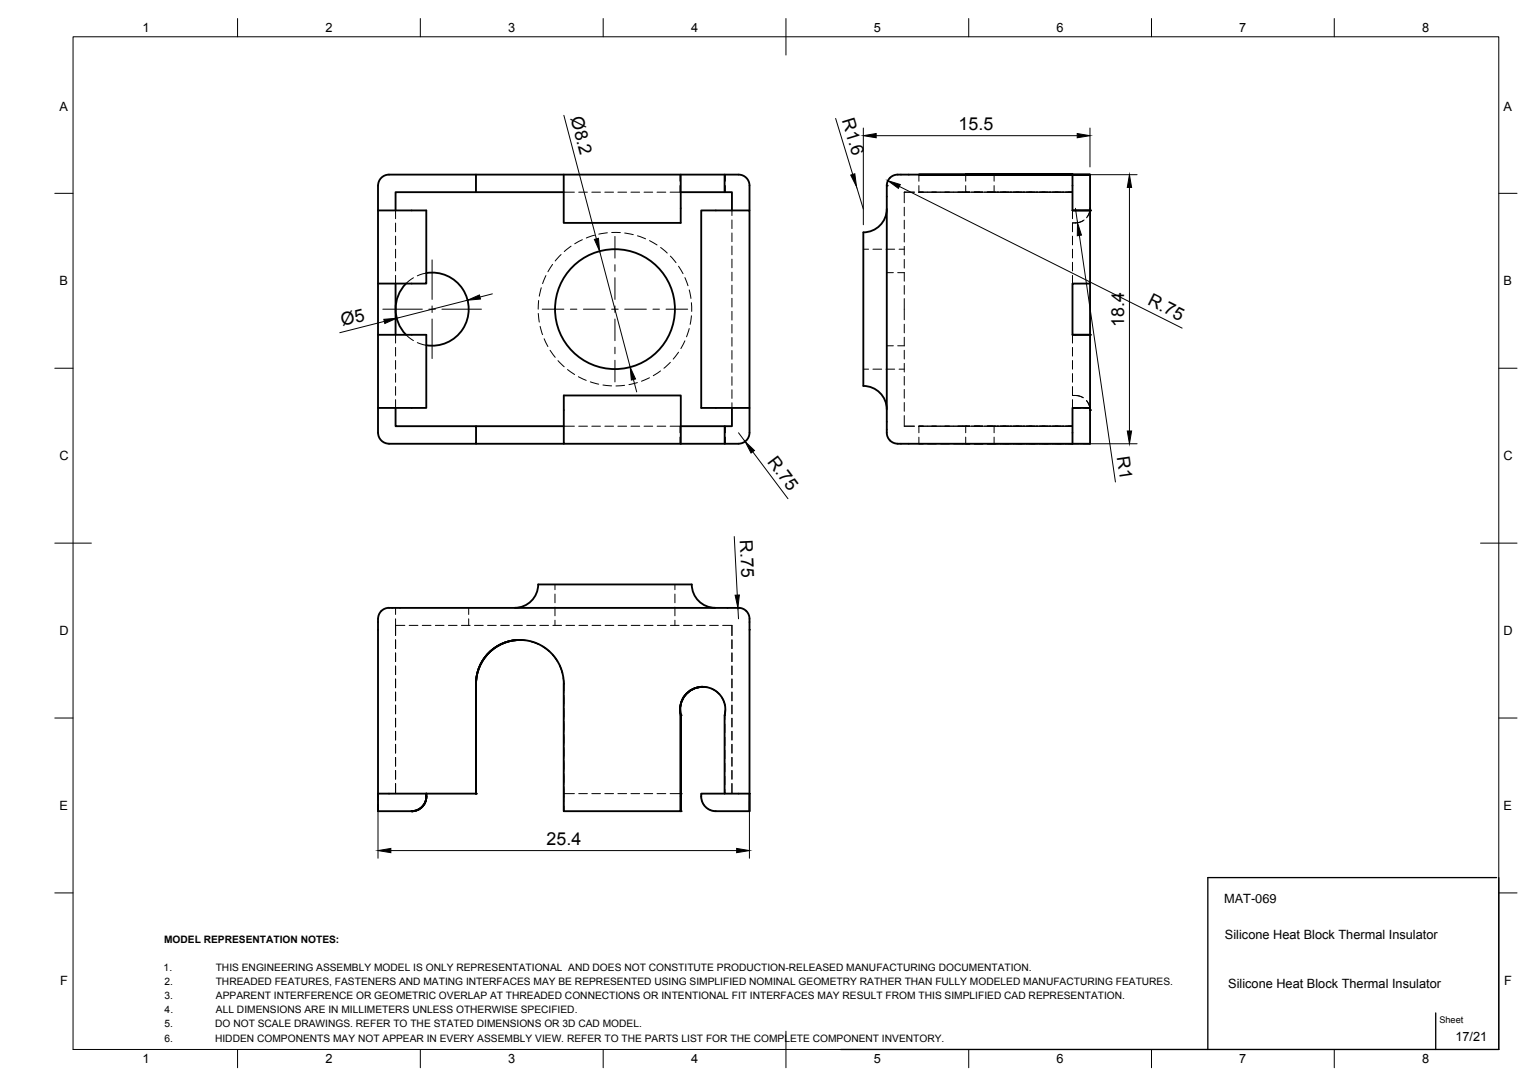
ISO-10303-21;
HEADER;
/* Generated by software containing ST-Developer
 * from STEP Tools, Inc. (www.steptools.com) 
 */

FILE_DESCRIPTION(
/* description */ ('CAx-IF Rec.Pracs.---Representation and Presentation of Product Manufa
cturing Information (PMI)---4.0---2014-10-13'),
/* implementation_level */ '2;1');

FILE_NAME(
/* name */ 'Silicone Heat Block Thermal Insulator.step',
/* time_stamp */ '2026-10-24T15:08:39-07:00',
/* author */ (''),
/* organization */ (''),
/* preprocessor_version */ 'ST-DEVELOPER v20.2',
/* originating_system */ 'Autodesk Translation Framework v15.17.0.0',
/* authorisation */ '');

FILE_SCHEMA (('AP242_MANAGED_MODEL_BASED_3D_ENGINEERING_MIM_LF { 1 0 10303 442 2 1 4 }'));
ENDSEC;

DATA;
#10=MECHANICAL_DESIGN_GEOMETRIC_PRESENTATION_REPRESENTATION('',(#834),#50081);
#115=B_SPLINE_SURFACE_WITH_KNOTS('',3,3,((#44428,#44429,#44430,#44431,#44432,
#44433),(#44434,#44435,#44436,#44437,#44438,#44439),(#44440,#44441,#44442,
#44443,#44444,#44445),(#44446,#44447,#44448,#44449,#44450,#44451),(#44452,
#44453,#44454,#44455,#44456,#44457),(#44458,#44459,#44460,#44461,#44462,
#44463)),.UNSPECIFIED.,.F.,.F.,.F.,(4,1,1,4),(4,1,1,4),(0.,0.333333333333333,
0.666666666666667,1.00005609897907),(-5.60989790777921E-5,0.333333333333333,
0.666666666666667,1.00005609897908),.UNSPECIFIED.);
#116=B_SPLINE_SURFACE_WITH_KNOTS('',3,3,((#44482,#44483,#44484,#44485,#44486,
#44487),(#44488,#44489,#44490,#44491,#44492,#44493),(#44494,#44495,#44496,
#44497,#44498,#44499),(#44500,#44501,#44502,#44503,#44504,#44505),(#44506,
#44507,#44508,#44509,#44510,#44511),(#44512,#44513,#44514,#44515,#44516,
#44517)),.UNSPECIFIED.,.F.,.F.,.F.,(4,1,1,4),(4,1,1,4),(-5.60989790420212E-5,
0.333333333333333,0.666666666666667,1.00005609897904),(0.,0.333333333333333,
0.666666666666667,1.00005609897904),.UNSPECIFIED.);
#117=B_SPLINE_SURFACE_WITH_KNOTS('',3,3,((#44528,#44529,#44530,#44531,#44532,
#44533),(#44534,#44535,#44536,#44537,#44538,#44539),(#44540,#44541,#44542,
#44543,#44544,#44545),(#44546,#44547,#44548,#44549,#44550,#44551),(#44552,
#44553,#44554,#44555,#44556,#44557),(#44558,#44559,#44560,#44561,#44562,
#44563)),.UNSPECIFIED.,.F.,.F.,.F.,(4,1,1,4),(4,1,1,4),(0.,0.333333333333333,
0.666666666666667,1.00005609897908),(-5.60989790915146E-5,0.333333333333333,
0.666666666666667,1.00005609897909),.UNSPECIFIED.);
#118=B_SPLINE_SURFACE_WITH_KNOTS('',3,3,((#44574,#44575,#44576,#44577,#44578,
#44579),(#44580,#44581,#44582,#44583,#44584,#44585),(#44586,#44587,#44588,
#44589,#44590,#44591),(#44592,#44593,#44594,#44595,#44596,#44597),(#44598,
#44599,#44600,#44601,#44602,#44603),(#44604,#44605,#44606,#44607,#44608,
#44609)),.UNSPECIFIED.,.F.,.F.,.F.,(4,1,1,4),(4,1,1,4),(-5.60989790792135E-5,
0.333333333333333,0.666666666666667,1.00005609897908),(0.,0.333333333333333,
0.666666666666667,1.00005609897907),.UNSPECIFIED.);
#119=B_SPLINE_SURFACE_WITH_KNOTS('',3,3,((#44620,#44621,#44622,#44623,#44624,
#44625),(#44626,#44627,#44628,#44629,#44630,#44631),(#44632,#44633,#44634,
#44635,#44636,#44637),(#44638,#44639,#44640,#44641,#44642,#44643),(#44644,
#44645,#44646,#44647,#44648,#44649),(#44650,#44651,#44652,#44653,#44654,
#44655)),.UNSPECIFIED.,.F.,.F.,.F.,(4,1,1,4),(4,1,1,4),(0.,0.333333333333333,
0.666666666666667,1.00005609897905),(-5.60989790491253E-5,0.333333333333333,
0.666666666666667,1.00005609897905),.UNSPECIFIED.);
#120=B_SPLINE_SURFACE_WITH_KNOTS('',3,3,((#44666,#44667,#44668,#44669,#44670,
#44671),(#44672,#44673,#44674,#44675,#44676,#44677),(#44678,#44679,#44680,
#44681,#44682,#44683),(#44684,#44685,#44686,#44687,#44688,#44689),(#44690,
#44691,#44692,#44693,#44694,#44695),(#44696,#44697,#44698,#44699,#44700,
#44701)),.UNSPECIFIED.,.F.,.F.,.F.,(4,1,1,4),(4,1,1,4),(0.,0.333333333333333,
0.666666666666667,1.00005609897395),(-5.60989810489178E-5,0.333333333333333,
0.666666666666667,1.00005609898105),.UNSPECIFIED.);
#121=B_SPLINE_SURFACE_WITH_KNOTS('',3,3,((#44720,#44721,#44722,#44723,#44724,
#44725),(#44726,#44727,#44728,#44729,#44730,#44731),(#44732,#44733,#44734,
#44735,#44736,#44737),(#44738,#44739,#44740,#44741,#44742,#44743),(#44744,
#44745,#44746,#44747,#44748,#44749),(#44750,#44751,#44752,#44753,#44754,
#44755)),.UNSPECIFIED.,.F.,.F.,.F.,(4,1,1,4),(4,1,1,4),(-5.60989793261701E-5,
0.333333333333333,0.666666666666667,1.00005609897933),(0.,0.333333333333333,
0.666666666666667,1.00005609896406),.UNSPECIFIED.);
#122=B_SPLINE_SURFACE_WITH_KNOTS('',3,3,((#44766,#44767,#44768,#44769,#44770,
#44771),(#44772,#44773,#44774,#44775,#44776,#44777),(#44778,#44779,#44780,
#44781,#44782,#44783),(#44784,#44785,#44786,#44787,#44788,#44789),(#44790,
#44791,#44792,#44793,#44794,#44795),(#44796,#44797,#44798,#44799,#44800,
#44801)),.UNSPECIFIED.,.F.,.F.,.F.,(4,1,1,4),(4,1,1,4),(0.,0.333333333333333,
0.666666666666667,1.00005609897906),(-5.60989790758371E-5,0.333333333333333,
0.666666666666667,1.00005609897907),.UNSPECIFIED.);
#123=B_SPLINE_SURFACE_WITH_KNOTS('',3,3,((#44812,#44813,#44814,#44815,#44816,
#44817),(#44818,#44819,#44820,#44821,#44822,#44823),(#44824,#44825,#44826,
#44827,#44828,#44829),(#44830,#44831,#44832,#44833,#44834,#44835),(#44836,
#44837,#44838,#44839,#44840,#44841),(#44842,#44843,#44844,#44845,#44846,
#44847)),.UNSPECIFIED.,.F.,.F.,.F.,(4,1,1,4),(4,1,1,4),(-5.60989790925808E-5,
0.333333333333333,0.666666666666667,1.00005609897909),(0.,0.333333333333333,
0.666666666666667,1.00005609897908),.UNSPECIFIED.);
#124=B_SPLINE_SURFACE_WITH_KNOTS('',3,3,((#44858,#44859,#44860,#44861,#44862,
#44863),(#44864,#44865,#44866,#44867,#44868,#44869),(#44870,#44871,#44872,
#44873,#44874,#44875),(#44876,#44877,#44878,#44879,#44880,#44881),(#44882,
#44883,#44884,#44885,#44886,#44887),(#44888,#44889,#44890,#44891,#44892,
#44893)),.UNSPECIFIED.,.F.,.F.,.F.,(4,1,1,4),(4,1,1,4),(0.,0.333333333333333,
0.666666666666667,1.00005609896405),(-5.60989793186213E-5,0.333333333333333,
0.666666666666667,1.00005609897932),.UNSPECIFIED.);
#125=B_SPLINE_SURFACE_WITH_KNOTS('',3,3,((#44904,#44905,#44906,#44907,#44908,
#44909),(#44910,#44911,#44912,#44913,#44914,#44915),(#44916,#44917,#44918,
#44919,#44920,#44921),(#44922,#44923,#44924,#44925,#44926,#44927),(#44928,
#44929,#44930,#44931,#44932,#44933),(#44934,#44935,#44936,#44937,#44938,
#44939)),.UNSPECIFIED.,.F.,.F.,.F.,(4,1,1,4),(4,1,1,4),(0.,0.333333333333333,
0.666666666666667,1.00005609896408),(-5.60989793518835E-5,0.333333333333333,
0.666666666666667,1.00005609897935),.UNSPECIFIED.);
#126=B_SPLINE_SURFACE_WITH_KNOTS('',3,3,((#44958,#44959,#44960,#44961,#44962,
#44963),(#44964,#44965,#44966,#44967,#44968,#44969),(#44970,#44971,#44972,
#44973,#44974,#44975),(#44976,#44977,#44978,#44979,#44980,#44981),(#44982,
#44983,#44984,#44985,#44986,#44987),(#44988,#44989,#44990,#44991,#44992,
#44993)),.UNSPECIFIED.,.F.,.F.,.F.,(4,1,1,4),(4,1,1,4),(-5.60989810425424E-5,
0.333333333333333,0.666666666666667,1.00005609898105),(0.,0.333333333333333,
0.666666666666667,1.00005609897395),.UNSPECIFIED.);
#127=B_SPLINE_SURFACE_WITH_KNOTS('',3,3,((#45004,#45005,#45006,#45007,#45008,
#45009),(#45010,#45011,#45012,#45013,#45014,#45015),(#45016,#45017,#45018,
#45019,#45020,#45021),(#45022,#45023,#45024,#45025,#45026,#45027),(#45028,
#45029,#45030,#45031,#45032,#45033),(#45034,#45035,#45036,#45037,#45038,
#45039)),.UNSPECIFIED.,.F.,.F.,.F.,(4,1,1,4),(4,1,1,4),(0.,0.333333333333333,
0.666666666666667,1.00005609897391),(-5.60989809954259E-5,0.333333333333333,
0.666666666666667,1.000056098981),.UNSPECIFIED.);
#128=B_SPLINE_SURFACE_WITH_KNOTS('',3,3,((#45050,#45051,#45052,#45053,#45054,
#45055),(#45056,#45057,#45058,#45059,#45060,#45061),(#45062,#45063,#45064,
#45065,#45066,#45067),(#45068,#45069,#45070,#45071,#45072,#45073),(#45074,
#45075,#45076,#45077,#45078,#45079),(#45080,#45081,#45082,#45083,#45084,
#45085)),.UNSPECIFIED.,.F.,.F.,.F.,(4,1,1,4),(4,1,1,4),(-5.60989793233286E-5,
0.333333333333333,0.666666666666667,1.00005609897932),(0.,0.333333333333333,
0.666666666666667,1.00005609896406),.UNSPECIFIED.);
#129=B_SPLINE_SURFACE_WITH_KNOTS('',3,3,((#45096,#45097,#45098,#45099,#45100,
#45101),(#45102,#45103,#45104,#45105,#45106,#45107),(#45108,#45109,#45110,
#45111,#45112,#45113),(#45114,#45115,#45116,#45117,#45118,#45119),(#45120,
#45121,#45122,#45123,#45124,#45125),(#45126,#45127,#45128,#45129,#45130,
#45131)),.UNSPECIFIED.,.F.,.F.,.F.,(4,1,1,4),(4,1,1,4),(0.,0.333333333333333,
0.666666666666667,1.0000560989791),(-5.60989791002414E-5,0.333333333333333,
0.666666666666667,1.0000560989791),.UNSPECIFIED.);
#130=B_SPLINE_SURFACE_WITH_KNOTS('',3,3,((#45142,#45143,#45144,#45145,#45146,
#45147),(#45148,#45149,#45150,#45151,#45152,#45153),(#45154,#45155,#45156,
#45157,#45158,#45159),(#45160,#45161,#45162,#45163,#45164,#45165),(#45166,
#45167,#45168,#45169,#45170,#45171),(#45172,#45173,#45174,#45175,#45176,
#45177)),.UNSPECIFIED.,.F.,.F.,.F.,(4,1,1,4),(4,1,1,4),(0.,0.333333333333333,
0.666666666666667,1.00005609896409),(-5.60989793533921E-5,0.333333333333333,
0.666666666666667,1.00005609897935),.UNSPECIFIED.);
#131=B_SPLINE_SURFACE_WITH_KNOTS('',3,3,((#45196,#45197,#45198,#45199,#45200,
#45201),(#45202,#45203,#45204,#45205,#45206,#45207),(#45208,#45209,#45210,
#45211,#45212,#45213),(#45214,#45215,#45216,#45217,#45218,#45219),(#45220,
#45221,#45222,#45223,#45224,#45225),(#45226,#45227,#45228,#45229,#45230,
#45231)),.UNSPECIFIED.,.F.,.F.,.F.,(4,1,1,4),(4,1,1,4),(-5.60989810493619E-5,
0.333333333333333,0.666666666666667,1.00005609898105),(0.,0.333333333333333,
0.666666666666667,1.00005609897395),.UNSPECIFIED.);
#132=B_SPLINE_SURFACE_WITH_KNOTS('',3,3,((#45242,#45243,#45244,#45245,#45246,
#45247),(#45248,#45249,#45250,#45251,#45252,#45253),(#45254,#45255,#45256,
#45257,#45258,#45259),(#45260,#45261,#45262,#45263,#45264,#45265),(#45266,
#45267,#45268,#45269,#45270,#45271),(#45272,#45273,#45274,#45275,#45276,
#45277)),.UNSPECIFIED.,.F.,.F.,.F.,(4,1,1,4),(4,1,1,4),(0.,0.333333333333333,
0.666666666666667,1.00005609895074),(-5.60989812701836E-5,0.333333333333333,
0.666666666666667,1.00005609898127),.UNSPECIFIED.);
#133=B_SPLINE_SURFACE_WITH_KNOTS('',3,3,((#45288,#45289,#45290,#45291,#45292,
#45293),(#45294,#45295,#45296,#45297,#45298,#45299),(#45300,#45301,#45302,
#45303,#45304,#45305),(#45306,#45307,#45308,#45309,#45310,#45311),(#45312,
#45313,#45314,#45315,#45316,#45317),(#45318,#45319,#45320,#45321,#45322,
#45323)),.UNSPECIFIED.,.F.,.F.,.F.,(4,1,1,4),(4,1,1,4),(-5.60989812733151E-5,
0.333333333333333,0.666666666666667,1.00005609898127),(0.,0.333333333333333,
0.666666666666667,1.00005609895075),.UNSPECIFIED.);
#134=B_SPLINE_SURFACE_WITH_KNOTS('',3,3,((#45334,#45335,#45336,#45337,#45338,
#45339),(#45340,#45341,#45342,#45343,#45344,#45345),(#45346,#45347,#45348,
#45349,#45350,#45351),(#45352,#45353,#45354,#45355,#45356,#45357),(#45358,
#45359,#45360,#45361,#45362,#45363),(#45364,#45365,#45366,#45367,#45368,
#45369)),.UNSPECIFIED.,.F.,.F.,.F.,(4,1,1,4),(4,1,1,4),(0.,0.333333333333333,
0.666666666666667,1.00005609897395),(-5.60989810488734E-5,0.333333333333333,
0.666666666666667,1.00005609898105),.UNSPECIFIED.);
#135=B_SPLINE_SURFACE_WITH_KNOTS('',3,3,((#45380,#45381,#45382,#45383,#45384,
#45385),(#45386,#45387,#45388,#45389,#45390,#45391),(#45392,#45393,#45394,
#45395,#45396,#45397),(#45398,#45399,#45400,#45401,#45402,#45403),(#45404,
#45405,#45406,#45407,#45408,#45409),(#45410,#45411,#45412,#45413,#45414,
#45415)),.UNSPECIFIED.,.F.,.F.,.F.,(4,1,1,4),(4,1,1,4),(-5.60989793545037E-5,
0.333333333333333,0.666666666666667,1.00005609897935),(0.,0.333333333333333,
0.666666666666667,1.00005609896409),.UNSPECIFIED.);
#136=B_SPLINE_SURFACE_WITH_KNOTS('',3,3,((#45425,#45426,#45427,#45428,#45429,
#45430),(#45431,#45432,#45433,#45434,#45435,#45436),(#45437,#45438,#45439,
#45440,#45441,#45442),(#45443,#45444,#45445,#45446,#45447,#45448),(#45449,
#45450,#45451,#45452,#45453,#45454),(#45455,#45456,#45457,#45458,#45459,
#45460)),.UNSPECIFIED.,.F.,.F.,.F.,(4,1,1,4),(4,1,1,4),(-5.60989790782798E-5,
0.333333333333333,0.666666666666667,1.00005609897908),(0.,0.333333333333333,
0.666666666666667,1.00005609897908),.UNSPECIFIED.);
#137=B_SPLINE_SURFACE_WITH_KNOTS('',3,3,((#45473,#45474,#45475,#45476,#45477,
#45478),(#45479,#45480,#45481,#45482,#45483,#45484),(#45485,#45486,#45487,
#45488,#45489,#45490),(#45491,#45492,#45493,#45494,#45495,#45496),(#45497,
#45498,#45499,#45500,#45501,#45502),(#45503,#45504,#45505,#45506,#45507,
#45508)),.UNSPECIFIED.,.F.,.F.,.F.,(4,1,1,4),(4,1,1,4),(-5.60989810261355E-5,
0.333333333333333,0.666666666666667,1.00005609898103),(0.,0.333333333333333,
0.666666666666667,1.00005609897399),.UNSPECIFIED.);
#138=B_SPLINE_SURFACE_WITH_KNOTS('',3,3,((#45518,#45519,#45520,#45521,#45522,
#45523),(#45524,#45525,#45526,#45527,#45528,#45529),(#45530,#45531,#45532,
#45533,#45534,#45535),(#45536,#45537,#45538,#45539,#45540,#45541),(#45542,
#45543,#45544,#45545,#45546,#45547),(#45548,#45549,#45550,#45551,#45552,
#45553)),.UNSPECIFIED.,.F.,.F.,.F.,(4,1,1,4),(4,1,1,4),(-5.6098979101063E-5,
0.333333333333333,0.666666666666667,1.0000560989791),(0.,0.333333333333333,
0.666666666666667,1.0000560989791),.UNSPECIFIED.);
#493=B_SPLINE_CURVE_WITH_KNOTS('',3,(#44466,#44467,#44468,#44469,#44470,
#44471),.UNSPECIFIED.,.F.,.F.,(4,1,1,4),(0.,0.333333333333333,0.666666666666667,
1.),.UNSPECIFIED.);
#494=B_SPLINE_CURVE_WITH_KNOTS('',3,(#44473,#44474,#44475,#44476,#44477,
#44478),.UNSPECIFIED.,.F.,.F.,(4,1,1,4),(0.,0.333333333333333,0.666666666666667,
1.),.UNSPECIFIED.);
#495=B_SPLINE_CURVE_WITH_KNOTS('',3,(#44519,#44520,#44521,#44522,#44523,
#44524),.UNSPECIFIED.,.F.,.F.,(4,1,1,4),(0.,0.333333333333333,0.666666666666667,
1.),.UNSPECIFIED.);
#496=B_SPLINE_CURVE_WITH_KNOTS('',3,(#44565,#44566,#44567,#44568,#44569,
#44570),.UNSPECIFIED.,.F.,.F.,(4,1,1,4),(0.,0.333333333333333,0.666666666666667,
1.),.UNSPECIFIED.);
#497=B_SPLINE_CURVE_WITH_KNOTS('',3,(#44611,#44612,#44613,#44614,#44615,
#44616),.UNSPECIFIED.,.F.,.F.,(4,1,1,4),(0.,0.333333333333333,0.666666666666667,
1.),.UNSPECIFIED.);
#498=B_SPLINE_CURVE_WITH_KNOTS('',3,(#44657,#44658,#44659,#44660,#44661,
#44662),.UNSPECIFIED.,.F.,.F.,(4,1,1,4),(0.,0.333333333333333,0.666666666666667,
1.),.UNSPECIFIED.);
#499=B_SPLINE_CURVE_WITH_KNOTS('',3,(#44704,#44705,#44706,#44707,#44708,
#44709),.UNSPECIFIED.,.F.,.F.,(4,1,1,4),(0.,0.333333333333333,0.666666666666667,
1.),.UNSPECIFIED.);
#500=B_SPLINE_CURVE_WITH_KNOTS('',3,(#44711,#44712,#44713,#44714,#44715,
#44716),.UNSPECIFIED.,.F.,.F.,(4,1,1,4),(0.,0.333333333333333,0.666666666666667,
1.),.UNSPECIFIED.);
#501=B_SPLINE_CURVE_WITH_KNOTS('',3,(#44757,#44758,#44759,#44760,#44761,
#44762),.UNSPECIFIED.,.F.,.F.,(4,1,1,4),(0.,0.333333333333333,0.666666666666667,
1.),.UNSPECIFIED.);
#502=B_SPLINE_CURVE_WITH_KNOTS('',3,(#44803,#44804,#44805,#44806,#44807,
#44808),.UNSPECIFIED.,.F.,.F.,(4,1,1,4),(0.,0.333333333333333,0.666666666666667,
1.),.UNSPECIFIED.);
#503=B_SPLINE_CURVE_WITH_KNOTS('',3,(#44849,#44850,#44851,#44852,#44853,
#44854),.UNSPECIFIED.,.F.,.F.,(4,1,1,4),(0.,0.333333333333333,0.666666666666667,
1.),.UNSPECIFIED.);
#504=B_SPLINE_CURVE_WITH_KNOTS('',3,(#44895,#44896,#44897,#44898,#44899,
#44900),.UNSPECIFIED.,.F.,.F.,(4,1,1,4),(0.,0.333333333333333,0.666666666666667,
1.),.UNSPECIFIED.);
#505=B_SPLINE_CURVE_WITH_KNOTS('',3,(#44942,#44943,#44944,#44945,#44946,
#44947),.UNSPECIFIED.,.F.,.F.,(4,1,1,4),(0.,0.333333333333333,0.666666666666667,
1.),.UNSPECIFIED.);
#506=B_SPLINE_CURVE_WITH_KNOTS('',3,(#44949,#44950,#44951,#44952,#44953,
#44954),.UNSPECIFIED.,.F.,.F.,(4,1,1,4),(0.,0.333333333333333,0.666666666666667,
1.),.UNSPECIFIED.);
#507=B_SPLINE_CURVE_WITH_KNOTS('',3,(#44995,#44996,#44997,#44998,#44999,
#45000),.UNSPECIFIED.,.F.,.F.,(4,1,1,4),(0.,0.333333333333333,0.666666666666667,
1.),.UNSPECIFIED.);
#508=B_SPLINE_CURVE_WITH_KNOTS('',3,(#45041,#45042,#45043,#45044,#45045,
#45046),.UNSPECIFIED.,.F.,.F.,(4,1,1,4),(0.,0.333333333333333,0.666666666666667,
1.),.UNSPECIFIED.);
#509=B_SPLINE_CURVE_WITH_KNOTS('',3,(#45087,#45088,#45089,#45090,#45091,
#45092),.UNSPECIFIED.,.F.,.F.,(4,1,1,4),(0.,0.333333333333333,0.666666666666667,
1.),.UNSPECIFIED.);
#510=B_SPLINE_CURVE_WITH_KNOTS('',3,(#45133,#45134,#45135,#45136,#45137,
#45138),.UNSPECIFIED.,.F.,.F.,(4,1,1,4),(0.,0.333333333333333,0.666666666666667,
1.),.UNSPECIFIED.);
#511=B_SPLINE_CURVE_WITH_KNOTS('',3,(#45180,#45181,#45182,#45183,#45184,
#45185),.UNSPECIFIED.,.F.,.F.,(4,1,1,4),(0.,0.333333333333333,0.666666666666667,
1.),.UNSPECIFIED.);
#512=B_SPLINE_CURVE_WITH_KNOTS('',3,(#45187,#45188,#45189,#45190,#45191,
#45192),.UNSPECIFIED.,.F.,.F.,(4,1,1,4),(0.,0.333333333333333,0.666666666666667,
1.),.UNSPECIFIED.);
#513=B_SPLINE_CURVE_WITH_KNOTS('',3,(#45233,#45234,#45235,#45236,#45237,
#45238),.UNSPECIFIED.,.F.,.F.,(4,1,1,4),(0.,0.333333333333333,0.666666666666667,
1.),.UNSPECIFIED.);
#514=B_SPLINE_CURVE_WITH_KNOTS('',3,(#45279,#45280,#45281,#45282,#45283,
#45284),.UNSPECIFIED.,.F.,.F.,(4,1,1,4),(0.,0.333333333333333,0.666666666666667,
1.),.UNSPECIFIED.);
#515=B_SPLINE_CURVE_WITH_KNOTS('',3,(#45325,#45326,#45327,#45328,#45329,
#45330),.UNSPECIFIED.,.F.,.F.,(4,1,1,4),(0.,0.333333333333333,0.666666666666667,
1.),.UNSPECIFIED.);
#516=B_SPLINE_CURVE_WITH_KNOTS('',3,(#45371,#45372,#45373,#45374,#45375,
#45376),.UNSPECIFIED.,.F.,.F.,(4,1,1,4),(0.,0.333333333333333,0.666666666666667,
1.),.UNSPECIFIED.);
#760=FACE_BOUND('',#2101,.T.);
#761=FACE_BOUND('',#2102,.T.);
#762=FACE_BOUND('',#2137,.T.);
#763=FACE_BOUND('',#2139,.T.);
#777=TOROIDAL_SURFACE('',#10859,0.00685,0.0016);
#794=SHAPE_REPRESENTATION_RELATIONSHIP('SRR','None',#50162,#814);
#814=ADVANCED_BREP_SHAPE_REPRESENTATION('',(#854),#50075);
#834=STYLED_ITEM('',(#50257),#854);
#854=MANIFOLD_SOLID_BREP('Body1',#9879);
#1038=PLANE('',#10809);
#1039=PLANE('',#10812);
#1040=PLANE('',#10813);
#1041=PLANE('',#10814);
#1042=PLANE('',#10815);
#1043=PLANE('',#10821);
#1044=PLANE('',#10822);
#1045=PLANE('',#10826);
#1046=PLANE('',#10827);
#1047=PLANE('',#10831);
#1048=PLANE('',#10832);
#1049=PLANE('',#10836);
#1050=PLANE('',#10837);
#1051=PLANE('',#10841);
#1052=PLANE('',#10842);
#1053=PLANE('',#10843);
#1054=PLANE('',#10844);
#1055=PLANE('',#10845);
#1056=PLANE('',#10846);
#1057=PLANE('',#10847);
#1058=PLANE('',#10848);
#1059=PLANE('',#10849);
#1060=PLANE('',#10850);
#1061=PLANE('',#10851);
#1062=PLANE('',#10852);
#1063=PLANE('',#10853);
#1064=PLANE('',#10854);
#1065=PLANE('',#10855);
#1066=PLANE('',#10856);
#1067=PLANE('',#10857);
#1068=PLANE('',#10858);
#1069=PLANE('',#10865);
#1070=PLANE('',#10866);
#1071=PLANE('',#10869);
#1072=PLANE('',#10870);
#1073=PLANE('',#10871);
#1074=PLANE('',#10874);
#1075=PLANE('',#10876);
#1076=PLANE('',#10877);
#1077=PLANE('',#10879);
#1078=PLANE('',#10883);
#1079=PLANE('',#10884);
#1080=PLANE('',#10888);
#1081=PLANE('',#10889);
#1082=PLANE('',#10890);
#1473=FACE_OUTER_BOUND('',#2064,.T.);
#1474=FACE_OUTER_BOUND('',#2065,.T.);
#1475=FACE_OUTER_BOUND('',#2066,.T.);
#1476=FACE_OUTER_BOUND('',#2067,.T.);
#1477=FACE_OUTER_BOUND('',#2068,.T.);
#1478=FACE_OUTER_BOUND('',#2069,.T.);
#1479=FACE_OUTER_BOUND('',#2070,.T.);
#1480=FACE_OUTER_BOUND('',#2071,.T.);
#1481=FACE_OUTER_BOUND('',#2072,.T.);
#1482=FACE_OUTER_BOUND('',#2073,.T.);
#1483=FACE_OUTER_BOUND('',#2074,.T.);
#1484=FACE_OUTER_BOUND('',#2075,.T.);
#1485=FACE_OUTER_BOUND('',#2076,.T.);
#1486=FACE_OUTER_BOUND('',#2077,.T.);
#1487=FACE_OUTER_BOUND('',#2078,.T.);
#1488=FACE_OUTER_BOUND('',#2079,.T.);
#1489=FACE_OUTER_BOUND('',#2080,.T.);
#1490=FACE_OUTER_BOUND('',#2081,.T.);
#1491=FACE_OUTER_BOUND('',#2082,.T.);
#1492=FACE_OUTER_BOUND('',#2083,.T.);
#1493=FACE_OUTER_BOUND('',#2084,.T.);
#1494=FACE_OUTER_BOUND('',#2085,.T.);
#1495=FACE_OUTER_BOUND('',#2086,.T.);
#1496=FACE_OUTER_BOUND('',#2087,.T.);
#1497=FACE_OUTER_BOUND('',#2088,.T.);
#1498=FACE_OUTER_BOUND('',#2089,.T.);
#1499=FACE_OUTER_BOUND('',#2090,.T.);
#1500=FACE_OUTER_BOUND('',#2091,.T.);
#1501=FACE_OUTER_BOUND('',#2092,.T.);
#1502=FACE_OUTER_BOUND('',#2093,.T.);
#1503=FACE_OUTER_BOUND('',#2094,.T.);
#1504=FACE_OUTER_BOUND('',#2095,.T.);
#1505=FACE_OUTER_BOUND('',#2096,.T.);
#1506=FACE_OUTER_BOUND('',#2097,.T.);
#1507=FACE_OUTER_BOUND('',#2098,.T.);
#1508=FACE_OUTER_BOUND('',#2099,.T.);
#1509=FACE_OUTER_BOUND('',#2100,.T.);
#1510=FACE_OUTER_BOUND('',#2103,.T.);
#1511=FACE_OUTER_BOUND('',#2104,.T.);
#1512=FACE_OUTER_BOUND('',#2105,.T.);
#1513=FACE_OUTER_BOUND('',#2106,.T.);
#1514=FACE_OUTER_BOUND('',#2107,.T.);
#1515=FACE_OUTER_BOUND('',#2108,.T.);
#1516=FACE_OUTER_BOUND('',#2109,.T.);
#1517=FACE_OUTER_BOUND('',#2110,.T.);
#1518=FACE_OUTER_BOUND('',#2111,.T.);
#1519=FACE_OUTER_BOUND('',#2112,.T.);
#1520=FACE_OUTER_BOUND('',#2113,.T.);
#1521=FACE_OUTER_BOUND('',#2114,.T.);
#1522=FACE_OUTER_BOUND('',#2115,.T.);
#1523=FACE_OUTER_BOUND('',#2116,.T.);
#1524=FACE_OUTER_BOUND('',#2117,.T.);
#1525=FACE_OUTER_BOUND('',#2118,.T.);
#1526=FACE_OUTER_BOUND('',#2119,.T.);
#1527=FACE_OUTER_BOUND('',#2120,.T.);
#1528=FACE_OUTER_BOUND('',#2121,.T.);
#1529=FACE_OUTER_BOUND('',#2122,.T.);
#1530=FACE_OUTER_BOUND('',#2123,.T.);
#1531=FACE_OUTER_BOUND('',#2124,.T.);
#1532=FACE_OUTER_BOUND('',#2125,.T.);
#1533=FACE_OUTER_BOUND('',#2126,.T.);
#1534=FACE_OUTER_BOUND('',#2127,.T.);
#1535=FACE_OUTER_BOUND('',#2128,.T.);
#1536=FACE_OUTER_BOUND('',#2129,.T.);
#1537=FACE_OUTER_BOUND('',#2130,.T.);
#1538=FACE_OUTER_BOUND('',#2131,.T.);
#1539=FACE_OUTER_BOUND('',#2132,.T.);
#1540=FACE_OUTER_BOUND('',#2133,.T.);
#1541=FACE_OUTER_BOUND('',#2134,.T.);
#1542=FACE_OUTER_BOUND('',#2135,.T.);
#1543=FACE_OUTER_BOUND('',#2136,.T.);
#1544=FACE_OUTER_BOUND('',#2138,.T.);
#1545=FACE_OUTER_BOUND('',#2140,.T.);
#1546=FACE_OUTER_BOUND('',#2141,.T.);
#1547=FACE_OUTER_BOUND('',#2142,.T.);
#1548=FACE_OUTER_BOUND('',#2143,.T.);
#1549=FACE_OUTER_BOUND('',#2144,.T.);
#1550=FACE_OUTER_BOUND('',#2145,.T.);
#1551=FACE_OUTER_BOUND('',#2146,.T.);
#1552=FACE_OUTER_BOUND('',#2147,.T.);
#1553=FACE_OUTER_BOUND('',#2148,.T.);
#1554=FACE_OUTER_BOUND('',#2149,.T.);
#1555=FACE_OUTER_BOUND('',#2150,.T.);
#1556=FACE_OUTER_BOUND('',#2151,.T.);
#1557=FACE_OUTER_BOUND('',#2152,.T.);
#1558=FACE_OUTER_BOUND('',#2153,.T.);
#1559=FACE_OUTER_BOUND('',#2154,.T.);
#1560=FACE_OUTER_BOUND('',#2155,.T.);
#1561=FACE_OUTER_BOUND('',#2156,.T.);
#2064=EDGE_LOOP('',(#8278,#8279,#8280,#8281));
#2065=EDGE_LOOP('',(#8282,#8283,#8284,#8285));
#2066=EDGE_LOOP('',(#8286,#8287,#8288,#8289));
#2067=EDGE_LOOP('',(#8290,#8291,#8292,#8293));
#2068=EDGE_LOOP('',(#8294,#8295,#8296,#8297));
#2069=EDGE_LOOP('',(#8298,#8299,#8300,#8301));
#2070=EDGE_LOOP('',(#8302,#8303,#8304,#8305));
#2071=EDGE_LOOP('',(#8306,#8307,#8308,#8309));
#2072=EDGE_LOOP('',(#8310,#8311,#8312,#8313));
#2073=EDGE_LOOP('',(#8314,#8315,#8316,#8317));
#2074=EDGE_LOOP('',(#8318,#8319,#8320,#8321));
#2075=EDGE_LOOP('',(#8322,#8323,#8324,#8325));
#2076=EDGE_LOOP('',(#8326,#8327,#8328,#8329));
#2077=EDGE_LOOP('',(#8330,#8331,#8332,#8333));
#2078=EDGE_LOOP('',(#8334,#8335,#8336,#8337));
#2079=EDGE_LOOP('',(#8338,#8339,#8340,#8341));
#2080=EDGE_LOOP('',(#8342,#8343,#8344,#8345));
#2081=EDGE_LOOP('',(#8346,#8347,#8348,#8349));
#2082=EDGE_LOOP('',(#8350,#8351,#8352,#8353));
#2083=EDGE_LOOP('',(#8354,#8355,#8356,#8357));
#2084=EDGE_LOOP('',(#8358,#8359,#8360,#8361));
#2085=EDGE_LOOP('',(#8362,#8363,#8364,#8365,#8366));
#2086=EDGE_LOOP('',(#8367,#8368,#8369,#8370));
#2087=EDGE_LOOP('',(#8371,#8372,#8373,#8374,#8375));
#2088=EDGE_LOOP('',(#8376,#8377,#8378,#8379,#8380,#8381));
#2089=EDGE_LOOP('',(#8382,#8383,#8384,#8385));
#2090=EDGE_LOOP('',(#8386,#8387,#8388,#8389,#8390));
#2091=EDGE_LOOP('',(#8391,#8392,#8393,#8394));
#2092=EDGE_LOOP('',(#8395,#8396,#8397,#8398,#8399));
#2093=EDGE_LOOP('',(#8400,#8401,#8402,#8403,#8404,#8405));
#2094=EDGE_LOOP('',(#8406,#8407,#8408,#8409,#8410,#8411));
#2095=EDGE_LOOP('',(#8412,#8413,#8414,#8415,#8416,#8417));
#2096=EDGE_LOOP('',(#8418,#8419,#8420,#8421,#8422,#8423,#8424,#8425,#8426,
#8427,#8428,#8429,#8430,#8431,#8432,#8433));
#2097=EDGE_LOOP('',(#8434,#8435,#8436,#8437,#8438,#8439,#8440));
#2098=EDGE_LOOP('',(#8441,#8442,#8443,#8444,#8445,#8446,#8447,#8448,#8449,
#8450,#8451,#8452,#8453,#8454,#8455,#8456));
#2099=EDGE_LOOP('',(#8457,#8458,#8459,#8460,#8461,#8462,#8463));
#2100=EDGE_LOOP('',(#8464,#8465,#8466,#8467,#8468,#8469,#8470,#8471,#8472,
#8473,#8474,#8475));
#2101=EDGE_LOOP('',(#8476));
#2102=EDGE_LOOP('',(#8477));
#2103=EDGE_LOOP('',(#8478,#8479,#8480,#8481));
#2104=EDGE_LOOP('',(#8482,#8483,#8484,#8485));
#2105=EDGE_LOOP('',(#8486,#8487,#8488,#8489,#8490,#8491));
#2106=EDGE_LOOP('',(#8492,#8493,#8494,#8495));
#2107=EDGE_LOOP('',(#8496,#8497,#8498,#8499));
#2108=EDGE_LOOP('',(#8500,#8501,#8502,#8503,#8504,#8505));
#2109=EDGE_LOOP('',(#8506,#8507,#8508,#8509));
#2110=EDGE_LOOP('',(#8510,#8511,#8512,#8513,#8514,#8515,#8516));
#2111=EDGE_LOOP('',(#8517,#8518,#8519,#8520));
#2112=EDGE_LOOP('',(#8521,#8522,#8523,#8524));
#2113=EDGE_LOOP('',(#8525,#8526,#8527,#8528,#8529,#8530,#8531));
#2114=EDGE_LOOP('',(#8532,#8533,#8534,#8535));
#2115=EDGE_LOOP('',(#8536,#8537,#8538,#8539));
#2116=EDGE_LOOP('',(#8540,#8541,#8542,#8543));
#2117=EDGE_LOOP('',(#8544,#8545,#8546,#8547,#8548,#8549));
#2118=EDGE_LOOP('',(#8550,#8551,#8552,#8553));
#2119=EDGE_LOOP('',(#8554,#8555,#8556,#8557));
#2120=EDGE_LOOP('',(#8558,#8559,#8560,#8561,#8562,#8563));
#2121=EDGE_LOOP('',(#8564,#8565,#8566,#8567,#8568,#8569,#8570));
#2122=EDGE_LOOP('',(#8571,#8572,#8573,#8574,#8575,#8576,#8577));
#2123=EDGE_LOOP('',(#8578,#8579,#8580,#8581));
#2124=EDGE_LOOP('',(#8582,#8583,#8584,#8585,#8586,#8587));
#2125=EDGE_LOOP('',(#8588,#8589,#8590,#8591));
#2126=EDGE_LOOP('',(#8592,#8593,#8594,#8595));
#2127=EDGE_LOOP('',(#8596,#8597,#8598,#8599));
#2128=EDGE_LOOP('',(#8600,#8601,#8602,#8603));
#2129=EDGE_LOOP('',(#8604,#8605,#8606,#8607));
#2130=EDGE_LOOP('',(#8608,#8609,#8610,#8611));
#2131=EDGE_LOOP('',(#8612,#8613,#8614,#8615,#8616,#8617));
#2132=EDGE_LOOP('',(#8618,#8619,#8620,#8621));
#2133=EDGE_LOOP('',(#8622,#8623,#8624,#8625));
#2134=EDGE_LOOP('',(#8626,#8627,#8628,#8629));
#2135=EDGE_LOOP('',(#8630,#8631,#8632,#8633));
#2136=EDGE_LOOP('',(#8634));
#2137=EDGE_LOOP('',(#8635));
#2138=EDGE_LOOP('',(#8636,#8637,#8638,#8639,#8640,#8641));
#2139=EDGE_LOOP('',(#8642));
#2140=EDGE_LOOP('',(#8643,#8644,#8645,#8646));
#2141=EDGE_LOOP('',(#8647,#8648,#8649,#8650,#8651,#8652));
#2142=EDGE_LOOP('',(#8653,#8654,#8655,#8656,#8657,#8658,#8659,#8660,#8661,
#8662,#8663,#8664));
#2143=EDGE_LOOP('',(#8665,#8666,#8667,#8668,#8669,#8670,#8671,#8672,#8673,
#8674,#8675,#8676));
#2144=EDGE_LOOP('',(#8677,#8678,#8679,#8680));
#2145=EDGE_LOOP('',(#8681,#8682,#8683,#8684));
#2146=EDGE_LOOP('',(#8685,#8686,#8687,#8688,#8689,#8690,#8691));
#2147=EDGE_LOOP('',(#8692,#8693,#8694,#8695));
#2148=EDGE_LOOP('',(#8696,#8697,#8698,#8699));
#2149=EDGE_LOOP('',(#8700,#8701,#8702,#8703,#8704,#8705,#8706,#8707,#8708));
#2150=EDGE_LOOP('',(#8709,#8710,#8711,#8712));
#2151=EDGE_LOOP('',(#8713,#8714,#8715,#8716));
#2152=EDGE_LOOP('',(#8717,#8718,#8719,#8720));
#2153=EDGE_LOOP('',(#8721,#8722,#8723,#8724));
#2154=EDGE_LOOP('',(#8725,#8726,#8727,#8728,#8729,#8730,#8731));
#2155=EDGE_LOOP('',(#8732,#8733,#8734,#8735,#8736,#8737,#8738,#8739,#8740,
#8741,#8742,#8743,#8744,#8745,#8746,#8747));
#2156=EDGE_LOOP('',(#8748,#8749,#8750,#8751,#8752,#8753,#8754,#8755,#8756,
#8757,#8758,#8759));
#2624=LINE('',#45423,#3202);
#2625=LINE('',#45424,#3203);
#2626=LINE('',#45468,#3204);
#2627=LINE('',#45469,#3205);
#2628=LINE('',#45471,#3206);
#2629=LINE('',#45472,#3207);
#2630=LINE('',#45516,#3208);
#2631=LINE('',#45517,#3209);
#2632=LINE('',#45561,#3210);
#2633=LINE('',#45562,#3211);
#2634=LINE('',#45564,#3212);
#2635=LINE('',#45565,#3213);
#2636=LINE('',#45567,#3214);
#2637=LINE('',#45568,#3215);
#2638=LINE('',#45570,#3216);
#2639=LINE('',#45571,#3217);
#2640=LINE('',#45574,#3218);
#2641=LINE('',#45576,#3219);
#2642=LINE('',#45580,#3220);
#2643=LINE('',#45582,#3221);
#2644=LINE('',#45584,#3222);
#2645=LINE('',#45588,#3223);
#2646=LINE('',#45589,#3224);
#2647=LINE('',#45592,#3225);
#2648=LINE('',#45594,#3226);
#2649=LINE('',#45596,#3227);
#2650=LINE('',#45598,#3228);
#2651=LINE('',#45599,#3229);
#2652=LINE('',#45602,#3230);
#2653=LINE('',#45604,#3231);
#2654=LINE('',#45606,#3232);
#2655=LINE('',#45608,#3233);
#2656=LINE('',#45610,#3234);
#2657=LINE('',#45612,#3235);
#2658=LINE('',#45614,#3236);
#2659=LINE('',#45615,#3237);
#2660=LINE('',#45618,#3238);
#2661=LINE('',#45620,#3239);
#2662=LINE('',#45622,#3240);
#2663=LINE('',#45624,#3241);
#2664=LINE('',#45625,#3242);
#2665=LINE('',#45636,#3243);
#2666=LINE('',#45639,#3244);
#2667=LINE('',#45641,#3245);
#2668=LINE('',#45642,#3246);
#2669=LINE('',#45645,#3247);
#2670=LINE('',#45647,#3248);
#2671=LINE('',#45648,#3249);
#2672=LINE('',#45654,#3250);
#2673=LINE('',#45657,#3251);
#2674=LINE('',#45659,#3252);
#2675=LINE('',#45660,#3253);
#2676=LINE('',#45663,#3254);
#2677=LINE('',#45664,#3255);
#2678=LINE('',#45670,#3256);
#2679=LINE('',#45673,#3257);
#2680=LINE('',#45675,#3258);
#2681=LINE('',#45677,#3259);
#2682=LINE('',#45679,#3260);
#2683=LINE('',#45681,#3261);
#2684=LINE('',#45682,#3262);
#2685=LINE('',#45684,#3263);
#2686=LINE('',#45690,#3264);
#2687=LINE('',#45693,#3265);
#2688=LINE('',#45696,#3266);
#2689=LINE('',#45698,#3267);
#2690=LINE('',#45700,#3268);
#2691=LINE('',#45702,#3269);
#2692=LINE('',#45704,#3270);
#2693=LINE('',#45705,#3271);
#2694=LINE('',#45708,#3272);
#2695=LINE('',#45709,#3273);
#2696=LINE('',#45715,#3274);
#2697=LINE('',#45718,#3275);
#2698=LINE('',#45721,#3276);
#2699=LINE('',#45723,#3277);
#2700=LINE('',#45724,#3278);
#2701=LINE('',#45727,#3279);
#2702=LINE('',#45729,#3280);
#2703=LINE('',#45731,#3281);
#2704=LINE('',#45732,#3282);
#2705=LINE('',#45735,#3283);
#2706=LINE('',#45737,#3284);
#2707=LINE('',#45738,#3285);
#2708=LINE('',#45740,#3286);
#2709=LINE('',#45743,#3287);
#2710=LINE('',#45744,#3288);
#2711=LINE('',#45746,#3289);
#2712=LINE('',#45748,#3290);
#2713=LINE('',#45750,#3291);
#2714=LINE('',#45752,#3292);
#2715=LINE('',#45753,#3293);
#2716=LINE('',#45756,#3294);
#2717=LINE('',#45758,#3295);
#2718=LINE('',#45759,#3296);
#2719=LINE('',#45760,#3297);
#2720=LINE('',#45763,#3298);
#2721=LINE('',#45764,#3299);
#2722=LINE('',#45766,#3300);
#2723=LINE('',#45768,#3301);
#2724=LINE('',#45771,#3302);
#2725=LINE('',#45772,#3303);
#2726=LINE('',#45775,#3304);
#2727=LINE('',#45776,#3305);
#2728=LINE('',#45779,#3306);
#2729=LINE('',#45780,#3307);
#2730=LINE('',#45782,#3308);
#2731=LINE('',#45784,#3309);
#2732=LINE('',#45785,#3310);
#2733=LINE('',#45787,#3311);
#2734=LINE('',#45791,#3312);
#2735=LINE('',#45792,#3313);
#2736=LINE('',#45795,#3314);
#2737=LINE('',#45796,#3315);
#2738=LINE('',#45805,#3316);
#2739=LINE('',#45812,#3317);
#2740=LINE('',#45814,#3318);
#2741=LINE('',#45816,#3319);
#2742=LINE('',#45818,#3320);
#2743=LINE('',#45819,#3321);
#2744=LINE('',#45821,#3322);
#2745=LINE('',#45823,#3323);
#2746=LINE('',#45824,#3324);
#2747=LINE('',#45828,#3325);
#2748=LINE('',#45831,#3326);
#2749=LINE('',#45832,#3327);
#2750=LINE('',#45834,#3328);
#2751=LINE('',#45837,#3329);
#2752=LINE('',#45840,#3330);
#2753=LINE('',#45842,#3331);
#2754=LINE('',#45845,#3332);
#2755=LINE('',#45851,#3333);
#2756=LINE('',#45853,#3334);
#2757=LINE('',#45854,#3335);
#2758=LINE('',#45857,#3336);
#2759=LINE('',#45859,#3337);
#2760=LINE('',#45860,#3338);
#2761=LINE('',#45866,#3339);
#2762=LINE('',#45868,#3340);
#2763=LINE('',#45869,#3341);
#3202=VECTOR('',#12790,1.);
#3203=VECTOR('',#12791,1.);
#3204=VECTOR('',#12800,1.);
#3205=VECTOR('',#12801,1.);
#3206=VECTOR('',#12804,1.);
#3207=VECTOR('',#12805,1.);
#3208=VECTOR('',#12814,1.);
#3209=VECTOR('',#12815,1.);
#3210=VECTOR('',#12824,1.);
#3211=VECTOR('',#12825,1.);
#3212=VECTOR('',#12828,1.);
#3213=VECTOR('',#12829,1.);
#3214=VECTOR('',#12832,1.);
#3215=VECTOR('',#12833,1.);
#3216=VECTOR('',#12836,1.);
#3217=VECTOR('',#12837,1.);
#3218=VECTOR('',#12840,1.);
#3219=VECTOR('',#12841,1.);
#3220=VECTOR('',#12844,1.);
#3221=VECTOR('',#12845,1.);
#3222=VECTOR('',#12846,1.);
#3223=VECTOR('',#12849,1.);
#3224=VECTOR('',#12850,1.);
#3225=VECTOR('',#12853,1.);
#3226=VECTOR('',#12854,1.);
#3227=VECTOR('',#12855,1.);
#3228=VECTOR('',#12856,1.);
#3229=VECTOR('',#12857,1.);
#3230=VECTOR('',#12860,1.);
#3231=VECTOR('',#12861,1.);
#3232=VECTOR('',#12862,1.);
#3233=VECTOR('',#12863,1.);
#3234=VECTOR('',#12864,1.);
#3235=VECTOR('',#12865,1.);
#3236=VECTOR('',#12866,1.);
#3237=VECTOR('',#12867,1.);
#3238=VECTOR('',#12870,1.);
#3239=VECTOR('',#12871,1.);
#3240=VECTOR('',#12872,1.);
#3241=VECTOR('',#12873,1.);
#3242=VECTOR('',#12874,1.);
#3243=VECTOR('',#12885,1.);
#3244=VECTOR('',#12888,1.);
#3245=VECTOR('',#12891,1.);
#3246=VECTOR('',#12892,1.);
#3247=VECTOR('',#12895,1.);
#3248=VECTOR('',#12896,1.);
#3249=VECTOR('',#12897,1.);
#3250=VECTOR('',#12902,1.);
#3251=VECTOR('',#12905,1.);
#3252=VECTOR('',#12908,1.);
#3253=VECTOR('',#12909,1.);
#3254=VECTOR('',#12912,1.);
#3255=VECTOR('',#12913,1.);
#3256=VECTOR('',#12918,1.);
#3257=VECTOR('',#12921,1.);
#3258=VECTOR('',#12924,1.);
#3259=VECTOR('',#12925,1.);
#3260=VECTOR('',#12926,1.);
#3261=VECTOR('',#12927,1.);
#3262=VECTOR('',#12928,1.);
#3263=VECTOR('',#12931,1.);
#3264=VECTOR('',#12936,1.);
#3265=VECTOR('',#12939,1.);
#3266=VECTOR('',#12942,1.);
#3267=VECTOR('',#12943,1.);
#3268=VECTOR('',#12944,1.);
#3269=VECTOR('',#12945,1.);
#3270=VECTOR('',#12946,1.);
#3271=VECTOR('',#12947,1.);
#3272=VECTOR('',#12950,1.);
#3273=VECTOR('',#12951,1.);
#3274=VECTOR('',#12956,1.);
#3275=VECTOR('',#12959,1.);
#3276=VECTOR('',#12962,1.);
#3277=VECTOR('',#12963,1.);
#3278=VECTOR('',#12964,1.);
#3279=VECTOR('',#12967,1.);
#3280=VECTOR('',#12968,1.);
#3281=VECTOR('',#12969,1.);
#3282=VECTOR('',#12970,1.);
#3283=VECTOR('',#12973,1.);
#3284=VECTOR('',#12974,1.);
#3285=VECTOR('',#12975,1.);
#3286=VECTOR('',#12978,1.);
#3287=VECTOR('',#12981,1.);
#3288=VECTOR('',#12982,1.);
#3289=VECTOR('',#12985,1.);
#3290=VECTOR('',#12986,1.);
#3291=VECTOR('',#12987,1.);
#3292=VECTOR('',#12988,1.);
#3293=VECTOR('',#12989,1.);
#3294=VECTOR('',#12992,1.);
#3295=VECTOR('',#12993,1.);
#3296=VECTOR('',#12994,1.);
#3297=VECTOR('',#12995,1.);
#3298=VECTOR('',#12998,1.);
#3299=VECTOR('',#12999,1.);
#3300=VECTOR('',#13002,1.);
#3301=VECTOR('',#13005,1.);
#3302=VECTOR('',#13008,1.);
#3303=VECTOR('',#13009,1.);
#3304=VECTOR('',#13012,1.);
#3305=VECTOR('',#13013,1.);
#3306=VECTOR('',#13016,1.);
#3307=VECTOR('',#13017,1.);
#3308=VECTOR('',#13020,1.);
#3309=VECTOR('',#13021,1.);
#3310=VECTOR('',#13022,1.);
#3311=VECTOR('',#13025,1.);
#3312=VECTOR('',#13030,1.);
#3313=VECTOR('',#13031,1.);
#3314=VECTOR('',#13034,1.);
#3315=VECTOR('',#13035,1.);
#3316=VECTOR('',#13046,0.0041);
#3317=VECTOR('',#13055,1.);
#3318=VECTOR('',#13056,1.);
#3319=VECTOR('',#13057,1.);
#3320=VECTOR('',#13058,1.);
#3321=VECTOR('',#13059,1.);
#3322=VECTOR('',#13062,0.0025);
#3323=VECTOR('',#13065,1.);
#3324=VECTOR('',#13066,1.);
#3325=VECTOR('',#13071,1.);
#3326=VECTOR('',#13074,1.);
#3327=VECTOR('',#13075,1.);
#3328=VECTOR('',#13076,1.);
#3329=VECTOR('',#13081,1.);
#3330=VECTOR('',#13086,1.);
#3331=VECTOR('',#13089,1.);
#3332=VECTOR('',#13094,1.);
#3333=VECTOR('',#13101,1.);
#3334=VECTOR('',#13104,1.);
#3335=VECTOR('',#13105,1.);
#3336=VECTOR('',#13108,1.);
#3337=VECTOR('',#13109,1.);
#3338=VECTOR('',#13110,1.);
#3339=VECTOR('',#13117,1.);
#3340=VECTOR('',#13120,1.);
#3341=VECTOR('',#13121,1.);
#3653=CIRCLE('',#10749,0.000749886741462474);
#3654=CIRCLE('',#10750,0.00075000000001);
#3655=CIRCLE('',#10751,0.00075000000001);
#3656=CIRCLE('',#10752,0.000749886741462474);
#3657=CIRCLE('',#10753,0.000749886741462474);
#3658=CIRCLE('',#10754,0.00075000000001);
#3659=CIRCLE('',#10755,0.00075000000001);
#3660=CIRCLE('',#10756,0.000749886741462474);
#3661=CIRCLE('',#10757,0.000749886741462474);
#3662=CIRCLE('',#10758,0.00075000000001);
#3663=CIRCLE('',#10759,0.000749886741462473);
#3664=CIRCLE('',#10760,0.000750000000010001);
#3665=CIRCLE('',#10761,0.00075000000001);
#3666=CIRCLE('',#10762,0.000749886741462473);
#3667=CIRCLE('',#10763,0.000749886741462478);
#3668=CIRCLE('',#10764,0.00075000000001);
#3669=CIRCLE('',#10765,0.000750000000010002);
#3670=CIRCLE('',#10766,0.000749886741462478);
#3671=CIRCLE('',#10767,0.000749886741462476);
#3672=CIRCLE('',#10768,0.000750000000010002);
#3673=CIRCLE('',#10769,0.000749886741462477);
#3674=CIRCLE('',#10770,0.00075000000001);
#3675=CIRCLE('',#10771,0.00075000000001);
#3676=CIRCLE('',#10772,0.000749886741462477);
#3677=CIRCLE('',#10773,0.000749886741462475);
#3678=CIRCLE('',#10774,0.00075000000001);
#3679=CIRCLE('',#10775,0.000750000000010001);
#3680=CIRCLE('',#10776,0.000749886741462475);
#3681=CIRCLE('',#10777,0.000749886741462475);
#3682=CIRCLE('',#10778,0.000750000000010001);
#3683=CIRCLE('',#10779,0.000749886741462475);
#3684=CIRCLE('',#10780,0.000750000000010002);
#3685=CIRCLE('',#10781,0.00075000000001);
#3686=CIRCLE('',#10782,0.000749886741462475);
#3687=CIRCLE('',#10783,0.000749886741462478);
#3688=CIRCLE('',#10784,0.00075000000001);
#3689=CIRCLE('',#10785,0.00075000000001);
#3690=CIRCLE('',#10786,0.000749886741462478);
#3691=CIRCLE('',#10787,0.000749886741462473);
#3692=CIRCLE('',#10788,0.00075000000001);
#3693=CIRCLE('',#10789,0.000750000000010002);
#3694=CIRCLE('',#10790,0.000749886741462473);
#3695=CIRCLE('',#10792,0.000750000000014142);
#3696=CIRCLE('',#10793,0.00075000000001);
#3697=CIRCLE('',#10794,0.000749886741462475);
#3698=CIRCLE('',#10796,0.000750000000014142);
#3699=CIRCLE('',#10798,0.000750000000010001);
#3700=CIRCLE('',#10799,0.000749886741462476);
#3701=CIRCLE('',#10801,0.000750000000014142);
#3702=CIRCLE('',#10802,0.00075000000001);
#3703=CIRCLE('',#10803,0.000749886741462474);
#3704=CIRCLE('',#10805,0.000750000000014142);
#3705=CIRCLE('',#10810,0.00300000000001);
#3706=CIRCLE('',#10811,0.00155000000001);
#3707=CIRCLE('',#10816,0.00685000000001);
#3708=CIRCLE('',#10817,0.00250000000001);
#3709=CIRCLE('',#10819,0.00100000000001414);
#3710=CIRCLE('',#10820,0.00100000000001414);
#3711=CIRCLE('',#10824,0.00100000000001414);
#3712=CIRCLE('',#10825,0.00100000000001414);
#3713=CIRCLE('',#10829,0.00100000000001414);
#3714=CIRCLE('',#10830,0.00100000000001414);
#3715=CIRCLE('',#10834,0.00100000000001414);
#3716=CIRCLE('',#10835,0.00100000000001414);
#3717=CIRCLE('',#10839,0.00100000000001414);
#3718=CIRCLE('',#10840,0.00100000000001414);
#3719=CIRCLE('',#10860,0.0016);
#3720=CIRCLE('',#10861,0.00525000000001);
#3721=CIRCLE('',#10863,0.00410000000001);
#3722=CIRCLE('',#10864,0.00410000000001);
#3723=CIRCLE('',#10867,0.00250000000001);
#3724=CIRCLE('',#10872,0.00300000000001);
#3725=CIRCLE('',#10873,0.00155000000001);
#3726=CIRCLE('',#10881,0.00155000000001);
#3727=CIRCLE('',#10882,0.00155000000001);
#3728=CIRCLE('',#10886,0.00300000000001);
#3729=CIRCLE('',#10887,0.00300000000001);
#4487=VERTEX_POINT('',#44464);
#4488=VERTEX_POINT('',#44465);
#4489=VERTEX_POINT('',#44472);
#4490=VERTEX_POINT('',#44479);
#4491=VERTEX_POINT('',#44518);
#4492=VERTEX_POINT('',#44525);
#4493=VERTEX_POINT('',#44564);
#4494=VERTEX_POINT('',#44571);
#4495=VERTEX_POINT('',#44610);
#4496=VERTEX_POINT('',#44617);
#4497=VERTEX_POINT('',#44656);
#4498=VERTEX_POINT('',#44663);
#4499=VERTEX_POINT('',#44702);
#4500=VERTEX_POINT('',#44703);
#4501=VERTEX_POINT('',#44710);
#4502=VERTEX_POINT('',#44717);
#4503=VERTEX_POINT('',#44756);
#4504=VERTEX_POINT('',#44763);
#4505=VERTEX_POINT('',#44802);
#4506=VERTEX_POINT('',#44809);
#4507=VERTEX_POINT('',#44848);
#4508=VERTEX_POINT('',#44855);
#4509=VERTEX_POINT('',#44894);
#4510=VERTEX_POINT('',#44901);
#4511=VERTEX_POINT('',#44940);
#4512=VERTEX_POINT('',#44941);
#4513=VERTEX_POINT('',#44948);
#4514=VERTEX_POINT('',#44955);
#4515=VERTEX_POINT('',#44994);
#4516=VERTEX_POINT('',#45001);
#4517=VERTEX_POINT('',#45040);
#4518=VERTEX_POINT('',#45047);
#4519=VERTEX_POINT('',#45086);
#4520=VERTEX_POINT('',#45093);
#4521=VERTEX_POINT('',#45132);
#4522=VERTEX_POINT('',#45139);
#4523=VERTEX_POINT('',#45178);
#4524=VERTEX_POINT('',#45179);
#4525=VERTEX_POINT('',#45186);
#4526=VERTEX_POINT('',#45193);
#4527=VERTEX_POINT('',#45232);
#4528=VERTEX_POINT('',#45239);
#4529=VERTEX_POINT('',#45278);
#4530=VERTEX_POINT('',#45285);
#4531=VERTEX_POINT('',#45324);
#4532=VERTEX_POINT('',#45331);
#4533=VERTEX_POINT('',#45370);
#4534=VERTEX_POINT('',#45377);
#4535=VERTEX_POINT('',#45416);
#4536=VERTEX_POINT('',#45420);
#4537=VERTEX_POINT('',#45421);
#4538=VERTEX_POINT('',#45461);
#4539=VERTEX_POINT('',#45465);
#4540=VERTEX_POINT('',#45466);
#4541=VERTEX_POINT('',#45509);
#4542=VERTEX_POINT('',#45513);
#4543=VERTEX_POINT('',#45514);
#4544=VERTEX_POINT('',#45554);
#4545=VERTEX_POINT('',#45558);
#4546=VERTEX_POINT('',#45559);
#4547=VERTEX_POINT('',#45573);
#4548=VERTEX_POINT('',#45575);
#4549=VERTEX_POINT('',#45577);
#4550=VERTEX_POINT('',#45579);
#4551=VERTEX_POINT('',#45581);
#4552=VERTEX_POINT('',#45583);
#4553=VERTEX_POINT('',#45585);
#4554=VERTEX_POINT('',#45587);
#4555=VERTEX_POINT('',#45591);
#4556=VERTEX_POINT('',#45593);
#4557=VERTEX_POINT('',#45595);
#4558=VERTEX_POINT('',#45597);
#4559=VERTEX_POINT('',#45601);
#4560=VERTEX_POINT('',#45603);
#4561=VERTEX_POINT('',#45605);
#4562=VERTEX_POINT('',#45607);
#4563=VERTEX_POINT('',#45609);
#4564=VERTEX_POINT('',#45611);
#4565=VERTEX_POINT('',#45613);
#4566=VERTEX_POINT('',#45617);
#4567=VERTEX_POINT('',#45619);
#4568=VERTEX_POINT('',#45621);
#4569=VERTEX_POINT('',#45623);
#4570=VERTEX_POINT('',#45627);
#4571=VERTEX_POINT('',#45629);
#4572=VERTEX_POINT('',#45632);
#4573=VERTEX_POINT('',#45633);
#4574=VERTEX_POINT('',#45635);
#4575=VERTEX_POINT('',#45637);
#4576=VERTEX_POINT('',#45644);
#4577=VERTEX_POINT('',#45646);
#4578=VERTEX_POINT('',#45650);
#4579=VERTEX_POINT('',#45651);
#4580=VERTEX_POINT('',#45653);
#4581=VERTEX_POINT('',#45655);
#4582=VERTEX_POINT('',#45662);
#4583=VERTEX_POINT('',#45666);
#4584=VERTEX_POINT('',#45667);
#4585=VERTEX_POINT('',#45669);
#4586=VERTEX_POINT('',#45671);
#4587=VERTEX_POINT('',#45676);
#4588=VERTEX_POINT('',#45678);
#4589=VERTEX_POINT('',#45680);
#4590=VERTEX_POINT('',#45686);
#4591=VERTEX_POINT('',#45687);
#4592=VERTEX_POINT('',#45689);
#4593=VERTEX_POINT('',#45691);
#4594=VERTEX_POINT('',#45695);
#4595=VERTEX_POINT('',#45697);
#4596=VERTEX_POINT('',#45699);
#4597=VERTEX_POINT('',#45701);
#4598=VERTEX_POINT('',#45703);
#4599=VERTEX_POINT('',#45707);
#4600=VERTEX_POINT('',#45711);
#4601=VERTEX_POINT('',#45712);
#4602=VERTEX_POINT('',#45714);
#4603=VERTEX_POINT('',#45716);
#4604=VERTEX_POINT('',#45720);
#4605=VERTEX_POINT('',#45722);
#4606=VERTEX_POINT('',#45726);
#4607=VERTEX_POINT('',#45728);
#4608=VERTEX_POINT('',#45730);
#4609=VERTEX_POINT('',#45734);
#4610=VERTEX_POINT('',#45736);
#4611=VERTEX_POINT('',#45742);
#4612=VERTEX_POINT('',#45747);
#4613=VERTEX_POINT('',#45749);
#4614=VERTEX_POINT('',#45751);
#4615=VERTEX_POINT('',#45755);
#4616=VERTEX_POINT('',#45757);
#4617=VERTEX_POINT('',#45762);
#4618=VERTEX_POINT('',#45770);
#4619=VERTEX_POINT('',#45774);
#4620=VERTEX_POINT('',#45778);
#4621=VERTEX_POINT('',#45783);
#4622=VERTEX_POINT('',#45790);
#4623=VERTEX_POINT('',#45794);
#4624=VERTEX_POINT('',#45798);
#4625=VERTEX_POINT('',#45802);
#4626=VERTEX_POINT('',#45804);
#4627=VERTEX_POINT('',#45809);
#4628=VERTEX_POINT('',#45811);
#4629=VERTEX_POINT('',#45813);
#4630=VERTEX_POINT('',#45815);
#4631=VERTEX_POINT('',#45817);
#4632=VERTEX_POINT('',#45827);
#4633=VERTEX_POINT('',#45829);
#4634=VERTEX_POINT('',#45833);
#4635=VERTEX_POINT('',#45847);
#4636=VERTEX_POINT('',#45849);
#4637=VERTEX_POINT('',#45856);
#4638=VERTEX_POINT('',#45858);
#4639=VERTEX_POINT('',#45862);
#4640=VERTEX_POINT('',#45864);
#5792=EDGE_CURVE('',#4487,#4488,#493,.T.);
#5793=EDGE_CURVE('',#4487,#4489,#494,.T.);
#5794=EDGE_CURVE('',#4489,#4490,#3653,.T.);
#5795=EDGE_CURVE('',#4488,#4490,#3654,.T.);
#5796=EDGE_CURVE('',#4487,#4491,#495,.T.);
#5797=EDGE_CURVE('',#4492,#4491,#3655,.T.);
#5798=EDGE_CURVE('',#4492,#4489,#3656,.T.);
#5799=EDGE_CURVE('',#4487,#4493,#496,.T.);
#5800=EDGE_CURVE('',#4493,#4494,#3657,.T.);
#5801=EDGE_CURVE('',#4491,#4494,#3658,.T.);
#5802=EDGE_CURVE('',#4487,#4495,#497,.T.);
#5803=EDGE_CURVE('',#4496,#4495,#3659,.T.);
#5804=EDGE_CURVE('',#4496,#4493,#3660,.T.);
#5805=EDGE_CURVE('',#4487,#4497,#498,.T.);
#5806=EDGE_CURVE('',#4497,#4498,#3661,.T.);
#5807=EDGE_CURVE('',#4495,#4498,#3662,.T.);
#5808=EDGE_CURVE('',#4499,#4500,#499,.T.);
#5809=EDGE_CURVE('',#4499,#4501,#500,.T.);
#5810=EDGE_CURVE('',#4501,#4502,#3663,.T.);
#5811=EDGE_CURVE('',#4500,#4502,#3664,.T.);
#5812=EDGE_CURVE('',#4499,#4503,#501,.T.);
#5813=EDGE_CURVE('',#4504,#4503,#3665,.T.);
#5814=EDGE_CURVE('',#4504,#4501,#3666,.T.);
#5815=EDGE_CURVE('',#4499,#4505,#502,.T.);
#5816=EDGE_CURVE('',#4505,#4506,#3667,.T.);
#5817=EDGE_CURVE('',#4503,#4506,#3668,.T.);
#5818=EDGE_CURVE('',#4499,#4507,#503,.T.);
#5819=EDGE_CURVE('',#4508,#4507,#3669,.T.);
#5820=EDGE_CURVE('',#4508,#4505,#3670,.T.);
#5821=EDGE_CURVE('',#4499,#4509,#504,.T.);
#5822=EDGE_CURVE('',#4509,#4510,#3671,.T.);
#5823=EDGE_CURVE('',#4507,#4510,#3672,.T.);
#5824=EDGE_CURVE('',#4511,#4512,#505,.T.);
#5825=EDGE_CURVE('',#4511,#4513,#506,.T.);
#5826=EDGE_CURVE('',#4513,#4514,#3673,.T.);
#5827=EDGE_CURVE('',#4512,#4514,#3674,.T.);
#5828=EDGE_CURVE('',#4511,#4515,#507,.T.);
#5829=EDGE_CURVE('',#4516,#4515,#3675,.T.);
#5830=EDGE_CURVE('',#4516,#4513,#3676,.T.);
#5831=EDGE_CURVE('',#4511,#4517,#508,.T.);
#5832=EDGE_CURVE('',#4517,#4518,#3677,.T.);
#5833=EDGE_CURVE('',#4515,#4518,#3678,.T.);
#5834=EDGE_CURVE('',#4511,#4519,#509,.T.);
#5835=EDGE_CURVE('',#4520,#4519,#3679,.T.);
#5836=EDGE_CURVE('',#4520,#4517,#3680,.T.);
#5837=EDGE_CURVE('',#4511,#4521,#510,.T.);
#5838=EDGE_CURVE('',#4521,#4522,#3681,.T.);
#5839=EDGE_CURVE('',#4519,#4522,#3682,.T.);
#5840=EDGE_CURVE('',#4523,#4524,#511,.T.);
#5841=EDGE_CURVE('',#4523,#4525,#512,.T.);
#5842=EDGE_CURVE('',#4525,#4526,#3683,.T.);
#5843=EDGE_CURVE('',#4524,#4526,#3684,.T.);
#5844=EDGE_CURVE('',#4523,#4527,#513,.T.);
#5845=EDGE_CURVE('',#4528,#4527,#3685,.T.);
#5846=EDGE_CURVE('',#4528,#4525,#3686,.T.);
#5847=EDGE_CURVE('',#4523,#4529,#514,.T.);
#5848=EDGE_CURVE('',#4529,#4530,#3687,.T.);
#5849=EDGE_CURVE('',#4527,#4530,#3688,.T.);
#5850=EDGE_CURVE('',#4523,#4531,#515,.T.);
#5851=EDGE_CURVE('',#4532,#4531,#3689,.T.);
#5852=EDGE_CURVE('',#4532,#4529,#3690,.T.);
#5853=EDGE_CURVE('',#4523,#4533,#516,.T.);
#5854=EDGE_CURVE('',#4533,#4534,#3691,.T.);
#5855=EDGE_CURVE('',#4531,#4534,#3692,.T.);
#5856=EDGE_CURVE('',#4535,#4524,#3693,.T.);
#5857=EDGE_CURVE('',#4535,#4533,#3694,.T.);
#5858=EDGE_CURVE('',#4536,#4537,#3695,.T.);
#5859=EDGE_CURVE('',#4537,#4535,#2624,.T.);
#5860=EDGE_CURVE('',#4526,#4536,#2625,.T.);
#5861=EDGE_CURVE('',#4538,#4512,#3696,.T.);
#5862=EDGE_CURVE('',#4538,#4521,#3697,.T.);
#5863=EDGE_CURVE('',#4539,#4540,#3698,.T.);
#5864=EDGE_CURVE('',#4540,#4538,#2626,.T.);
#5865=EDGE_CURVE('',#4514,#4539,#2627,.T.);
#5866=EDGE_CURVE('',#4530,#4520,#2628,.T.);
#5867=EDGE_CURVE('',#4522,#4528,#2629,.T.);
#5868=EDGE_CURVE('',#4541,#4500,#3699,.T.);
#5869=EDGE_CURVE('',#4541,#4509,#3700,.T.);
#5870=EDGE_CURVE('',#4542,#4543,#3701,.T.);
#5871=EDGE_CURVE('',#4543,#4504,#2630,.T.);
#5872=EDGE_CURVE('',#4506,#4542,#2631,.T.);
#5873=EDGE_CURVE('',#4544,#4488,#3702,.T.);
#5874=EDGE_CURVE('',#4544,#4497,#3703,.T.);
#5875=EDGE_CURVE('',#4545,#4546,#3704,.T.);
#5876=EDGE_CURVE('',#4546,#4496,#2632,.T.);
#5877=EDGE_CURVE('',#4498,#4545,#2633,.T.);
#5878=EDGE_CURVE('',#4518,#4492,#2634,.T.);
#5879=EDGE_CURVE('',#4494,#4516,#2635,.T.);
#5880=EDGE_CURVE('',#4490,#4541,#2636,.T.);
#5881=EDGE_CURVE('',#4502,#4544,#2637,.T.);
#5882=EDGE_CURVE('',#4510,#4532,#2638,.T.);
#5883=EDGE_CURVE('',#4534,#4508,#2639,.T.);
#5884=EDGE_CURVE('',#4547,#4540,#2640,.T.);
#5885=EDGE_CURVE('',#4547,#4548,#2641,.T.);
#5886=EDGE_CURVE('',#4548,#4549,#3705,.T.);
#5887=EDGE_CURVE('',#4549,#4550,#2642,.T.);
#5888=EDGE_CURVE('',#4551,#4550,#2643,.T.);
#5889=EDGE_CURVE('',#4552,#4551,#2644,.T.);
#5890=EDGE_CURVE('',#4552,#4553,#3706,.T.);
#5891=EDGE_CURVE('',#4553,#4554,#2645,.T.);
#5892=EDGE_CURVE('',#4554,#4536,#2646,.T.);
#5893=EDGE_CURVE('',#4555,#4539,#2647,.T.);
#5894=EDGE_CURVE('',#4555,#4556,#2648,.T.);
#5895=EDGE_CURVE('',#4557,#4556,#2649,.T.);
#5896=EDGE_CURVE('',#4557,#4558,#2650,.T.);
#5897=EDGE_CURVE('',#4558,#4547,#2651,.T.);
#5898=EDGE_CURVE('',#4546,#4559,#2652,.T.);
#5899=EDGE_CURVE('',#4559,#4560,#2653,.T.);
#5900=EDGE_CURVE('',#4561,#4560,#2654,.T.);
#5901=EDGE_CURVE('',#4562,#4561,#2655,.T.);
#5902=EDGE_CURVE('',#4562,#4563,#2656,.T.);
#5903=EDGE_CURVE('',#4563,#4564,#2657,.T.);
#5904=EDGE_CURVE('',#4565,#4564,#2658,.T.);
#5905=EDGE_CURVE('',#4555,#4565,#2659,.T.);
#5906=EDGE_CURVE('',#4566,#4545,#2660,.T.);
#5907=EDGE_CURVE('',#4567,#4566,#2661,.T.);
#5908=EDGE_CURVE('',#4568,#4567,#2662,.T.);
#5909=EDGE_CURVE('',#4569,#4568,#2663,.T.);
#5910=EDGE_CURVE('',#4569,#4559,#2664,.T.);
#5911=EDGE_CURVE('',#4570,#4570,#3707,.T.);
#5912=EDGE_CURVE('',#4571,#4571,#3708,.T.);
#5913=EDGE_CURVE('',#4572,#4573,#3709,.T.);
#5914=EDGE_CURVE('',#4573,#4574,#2665,.T.);
#5915=EDGE_CURVE('',#4574,#4575,#3710,.T.);
#5916=EDGE_CURVE('',#4575,#4572,#2666,.T.);
#5917=EDGE_CURVE('',#4573,#4561,#2667,.T.);
#5918=EDGE_CURVE('',#4560,#4574,#2668,.T.);
#5919=EDGE_CURVE('',#4576,#4572,#2669,.T.);
#5920=EDGE_CURVE('',#4576,#4577,#2670,.T.);
#5921=EDGE_CURVE('',#4562,#4577,#2671,.T.);
#5922=EDGE_CURVE('',#4578,#4579,#3711,.T.);
#5923=EDGE_CURVE('',#4579,#4580,#2672,.T.);
#5924=EDGE_CURVE('',#4580,#4581,#3712,.T.);
#5925=EDGE_CURVE('',#4581,#4578,#2673,.T.);
#5926=EDGE_CURVE('',#4579,#4565,#2674,.T.);
#5927=EDGE_CURVE('',#4564,#4580,#2675,.T.);
#5928=EDGE_CURVE('',#4582,#4578,#2676,.T.);
#5929=EDGE_CURVE('',#4556,#4582,#2677,.T.);
#5930=EDGE_CURVE('',#4583,#4584,#3713,.T.);
#5931=EDGE_CURVE('',#4584,#4585,#2678,.T.);
#5932=EDGE_CURVE('',#4585,#4586,#3714,.T.);
#5933=EDGE_CURVE('',#4586,#4583,#2679,.T.);
#5934=EDGE_CURVE('',#4550,#4585,#2680,.T.);
#5935=EDGE_CURVE('',#4587,#4549,#2681,.T.);
#5936=EDGE_CURVE('',#4587,#4588,#2682,.T.);
#5937=EDGE_CURVE('',#4588,#4589,#2683,.T.);
#5938=EDGE_CURVE('',#4589,#4586,#2684,.T.);
#5939=EDGE_CURVE('',#4584,#4551,#2685,.T.);
#5940=EDGE_CURVE('',#4590,#4591,#3715,.T.);
#5941=EDGE_CURVE('',#4591,#4592,#2686,.T.);
#5942=EDGE_CURVE('',#4592,#4593,#3716,.T.);
#5943=EDGE_CURVE('',#4593,#4590,#2687,.T.);
#5944=EDGE_CURVE('',#4594,#4592,#2688,.T.);
#5945=EDGE_CURVE('',#4595,#4594,#2689,.T.);
#5946=EDGE_CURVE('',#4596,#4595,#2690,.T.);
#5947=EDGE_CURVE('',#4596,#4597,#2691,.T.);
#5948=EDGE_CURVE('',#4598,#4597,#2692,.T.);
#5949=EDGE_CURVE('',#4598,#4593,#2693,.T.);
#5950=EDGE_CURVE('',#4591,#4599,#2694,.T.);
#5951=EDGE_CURVE('',#4599,#4594,#2695,.T.);
#5952=EDGE_CURVE('',#4600,#4601,#3717,.T.);
#5953=EDGE_CURVE('',#4601,#4602,#2696,.T.);
#5954=EDGE_CURVE('',#4602,#4603,#3718,.T.);
#5955=EDGE_CURVE('',#4603,#4600,#2697,.T.);
#5956=EDGE_CURVE('',#4601,#4604,#2698,.T.);
#5957=EDGE_CURVE('',#4604,#4605,#2699,.T.);
#5958=EDGE_CURVE('',#4605,#4602,#2700,.T.);
#5959=EDGE_CURVE('',#4606,#4600,#2701,.T.);
#5960=EDGE_CURVE('',#4607,#4606,#2702,.T.);
#5961=EDGE_CURVE('',#4608,#4607,#2703,.T.);
#5962=EDGE_CURVE('',#4608,#4604,#2704,.T.);
#5963=EDGE_CURVE('',#4607,#4609,#2705,.T.);
#5964=EDGE_CURVE('',#4606,#4610,#2706,.T.);
#5965=EDGE_CURVE('',#4610,#4609,#2707,.T.);
#5966=EDGE_CURVE('',#4610,#4603,#2708,.T.);
#5967=EDGE_CURVE('',#4611,#4605,#2709,.T.);
#5968=EDGE_CURVE('',#4609,#4611,#2710,.T.);
#5969=EDGE_CURVE('',#4608,#4542,#2711,.T.);
#5970=EDGE_CURVE('',#4612,#4607,#2712,.T.);
#5971=EDGE_CURVE('',#4613,#4612,#2713,.T.);
#5972=EDGE_CURVE('',#4613,#4614,#2714,.T.);
#5973=EDGE_CURVE('',#4614,#4543,#2715,.T.);
#5974=EDGE_CURVE('',#4615,#4554,#2716,.T.);
#5975=EDGE_CURVE('',#4615,#4616,#2717,.T.);
#5976=EDGE_CURVE('',#4609,#4616,#2718,.T.);
#5977=EDGE_CURVE('',#4537,#4611,#2719,.T.);
#5978=EDGE_CURVE('',#4617,#4575,#2720,.T.);
#5979=EDGE_CURVE('',#4617,#4576,#2721,.T.);
#5980=EDGE_CURVE('',#4569,#4617,#2722,.T.);
#5981=EDGE_CURVE('',#4577,#4569,#2723,.T.);
#5982=EDGE_CURVE('',#4618,#4577,#2724,.T.);
#5983=EDGE_CURVE('',#4618,#4563,#2725,.T.);
#5984=EDGE_CURVE('',#4619,#4598,#2726,.T.);
#5985=EDGE_CURVE('',#4619,#4590,#2727,.T.);
#5986=EDGE_CURVE('',#4620,#4597,#2728,.T.);
#5987=EDGE_CURVE('',#4620,#4619,#2729,.T.);
#5988=EDGE_CURVE('',#4556,#4618,#2730,.T.);
#5989=EDGE_CURVE('',#4582,#4621,#2731,.T.);
#5990=EDGE_CURVE('',#4621,#4618,#2732,.T.);
#5991=EDGE_CURVE('',#4621,#4581,#2733,.T.);
#5992=EDGE_CURVE('',#4589,#4622,#2734,.T.);
#5993=EDGE_CURVE('',#4622,#4583,#2735,.T.);
#5994=EDGE_CURVE('',#4588,#4623,#2736,.T.);
#5995=EDGE_CURVE('',#4622,#4623,#2737,.T.);
#5996=EDGE_CURVE('',#4570,#4624,#3719,.T.);
#5997=EDGE_CURVE('',#4624,#4624,#3720,.T.);
#5998=EDGE_CURVE('',#4625,#4625,#3721,.T.);
#5999=EDGE_CURVE('',#4625,#4626,#2738,.T.);
#6000=EDGE_CURVE('',#4626,#4626,#3722,.T.);
#6001=EDGE_CURVE('',#4627,#4627,#3723,.T.);
#6002=EDGE_CURVE('',#4628,#4627,#2739,.T.);
#6003=EDGE_CURVE('',#4629,#4628,#2740,.T.);
#6004=EDGE_CURVE('',#4630,#4629,#2741,.T.);
#6005=EDGE_CURVE('',#4630,#4631,#2742,.T.);
#6006=EDGE_CURVE('',#4627,#4631,#2743,.T.);
#6007=EDGE_CURVE('',#4627,#4571,#2744,.T.);
#6008=EDGE_CURVE('',#4612,#4629,#2745,.T.);
#6009=EDGE_CURVE('',#4616,#4630,#2746,.T.);
#6010=EDGE_CURVE('',#4623,#4632,#2747,.T.);
#6011=EDGE_CURVE('',#4633,#4587,#3724,.T.);
#6012=EDGE_CURVE('',#4558,#4633,#2748,.T.);
#6013=EDGE_CURVE('',#4631,#4557,#2749,.T.);
#6014=EDGE_CURVE('',#4634,#4615,#2750,.T.);
#6015=EDGE_CURVE('',#4632,#4634,#3725,.T.);
#6016=EDGE_CURVE('',#4633,#4548,#2751,.T.);
#6017=EDGE_CURVE('',#4632,#4552,#2752,.T.);
#6018=EDGE_CURVE('',#4634,#4553,#2753,.T.);
#6019=EDGE_CURVE('',#4628,#4568,#2754,.T.);
#6020=EDGE_CURVE('',#4596,#4635,#3726,.T.);
#6021=EDGE_CURVE('',#4636,#4595,#3727,.T.);
#6022=EDGE_CURVE('',#4635,#4636,#2755,.T.);
#6023=EDGE_CURVE('',#4635,#4613,#2756,.T.);
#6024=EDGE_CURVE('',#4614,#4636,#2757,.T.);
#6025=EDGE_CURVE('',#4637,#4567,#2758,.T.);
#6026=EDGE_CURVE('',#4638,#4566,#2759,.T.);
#6027=EDGE_CURVE('',#4637,#4638,#2760,.T.);
#6028=EDGE_CURVE('',#4637,#4639,#3728,.T.);
#6029=EDGE_CURVE('',#4640,#4638,#3729,.T.);
#6030=EDGE_CURVE('',#4639,#4640,#2761,.T.);
#6031=EDGE_CURVE('',#4639,#4620,#2762,.T.);
#6032=EDGE_CURVE('',#4640,#4599,#2763,.T.);
#8278=ORIENTED_EDGE('',*,*,#5792,.F.);
#8279=ORIENTED_EDGE('',*,*,#5793,.T.);
#8280=ORIENTED_EDGE('',*,*,#5794,.T.);
#8281=ORIENTED_EDGE('',*,*,#5795,.F.);
#8282=ORIENTED_EDGE('',*,*,#5793,.F.);
#8283=ORIENTED_EDGE('',*,*,#5796,.T.);
#8284=ORIENTED_EDGE('',*,*,#5797,.F.);
#8285=ORIENTED_EDGE('',*,*,#5798,.T.);
#8286=ORIENTED_EDGE('',*,*,#5796,.F.);
#8287=ORIENTED_EDGE('',*,*,#5799,.T.);
#8288=ORIENTED_EDGE('',*,*,#5800,.T.);
#8289=ORIENTED_EDGE('',*,*,#5801,.F.);
#8290=ORIENTED_EDGE('',*,*,#5799,.F.);
#8291=ORIENTED_EDGE('',*,*,#5802,.T.);
#8292=ORIENTED_EDGE('',*,*,#5803,.F.);
#8293=ORIENTED_EDGE('',*,*,#5804,.T.);
#8294=ORIENTED_EDGE('',*,*,#5802,.F.);
#8295=ORIENTED_EDGE('',*,*,#5805,.T.);
#8296=ORIENTED_EDGE('',*,*,#5806,.T.);
#8297=ORIENTED_EDGE('',*,*,#5807,.F.);
#8298=ORIENTED_EDGE('',*,*,#5808,.F.);
#8299=ORIENTED_EDGE('',*,*,#5809,.T.);
#8300=ORIENTED_EDGE('',*,*,#5810,.T.);
#8301=ORIENTED_EDGE('',*,*,#5811,.F.);
#8302=ORIENTED_EDGE('',*,*,#5809,.F.);
#8303=ORIENTED_EDGE('',*,*,#5812,.T.);
#8304=ORIENTED_EDGE('',*,*,#5813,.F.);
#8305=ORIENTED_EDGE('',*,*,#5814,.T.);
#8306=ORIENTED_EDGE('',*,*,#5812,.F.);
#8307=ORIENTED_EDGE('',*,*,#5815,.T.);
#8308=ORIENTED_EDGE('',*,*,#5816,.T.);
#8309=ORIENTED_EDGE('',*,*,#5817,.F.);
#8310=ORIENTED_EDGE('',*,*,#5815,.F.);
#8311=ORIENTED_EDGE('',*,*,#5818,.T.);
#8312=ORIENTED_EDGE('',*,*,#5819,.F.);
#8313=ORIENTED_EDGE('',*,*,#5820,.T.);
#8314=ORIENTED_EDGE('',*,*,#5818,.F.);
#8315=ORIENTED_EDGE('',*,*,#5821,.T.);
#8316=ORIENTED_EDGE('',*,*,#5822,.T.);
#8317=ORIENTED_EDGE('',*,*,#5823,.F.);
#8318=ORIENTED_EDGE('',*,*,#5824,.F.);
#8319=ORIENTED_EDGE('',*,*,#5825,.T.);
#8320=ORIENTED_EDGE('',*,*,#5826,.T.);
#8321=ORIENTED_EDGE('',*,*,#5827,.F.);
#8322=ORIENTED_EDGE('',*,*,#5825,.F.);
#8323=ORIENTED_EDGE('',*,*,#5828,.T.);
#8324=ORIENTED_EDGE('',*,*,#5829,.F.);
#8325=ORIENTED_EDGE('',*,*,#5830,.T.);
#8326=ORIENTED_EDGE('',*,*,#5828,.F.);
#8327=ORIENTED_EDGE('',*,*,#5831,.T.);
#8328=ORIENTED_EDGE('',*,*,#5832,.T.);
#8329=ORIENTED_EDGE('',*,*,#5833,.F.);
#8330=ORIENTED_EDGE('',*,*,#5831,.F.);
#8331=ORIENTED_EDGE('',*,*,#5834,.T.);
#8332=ORIENTED_EDGE('',*,*,#5835,.F.);
#8333=ORIENTED_EDGE('',*,*,#5836,.T.);
#8334=ORIENTED_EDGE('',*,*,#5834,.F.);
#8335=ORIENTED_EDGE('',*,*,#5837,.T.);
#8336=ORIENTED_EDGE('',*,*,#5838,.T.);
#8337=ORIENTED_EDGE('',*,*,#5839,.F.);
#8338=ORIENTED_EDGE('',*,*,#5840,.F.);
#8339=ORIENTED_EDGE('',*,*,#5841,.T.);
#8340=ORIENTED_EDGE('',*,*,#5842,.T.);
#8341=ORIENTED_EDGE('',*,*,#5843,.F.);
#8342=ORIENTED_EDGE('',*,*,#5841,.F.);
#8343=ORIENTED_EDGE('',*,*,#5844,.T.);
#8344=ORIENTED_EDGE('',*,*,#5845,.F.);
#8345=ORIENTED_EDGE('',*,*,#5846,.T.);
#8346=ORIENTED_EDGE('',*,*,#5844,.F.);
#8347=ORIENTED_EDGE('',*,*,#5847,.T.);
#8348=ORIENTED_EDGE('',*,*,#5848,.T.);
#8349=ORIENTED_EDGE('',*,*,#5849,.F.);
#8350=ORIENTED_EDGE('',*,*,#5847,.F.);
#8351=ORIENTED_EDGE('',*,*,#5850,.T.);
#8352=ORIENTED_EDGE('',*,*,#5851,.F.);
#8353=ORIENTED_EDGE('',*,*,#5852,.T.);
#8354=ORIENTED_EDGE('',*,*,#5850,.F.);
#8355=ORIENTED_EDGE('',*,*,#5853,.T.);
#8356=ORIENTED_EDGE('',*,*,#5854,.T.);
#8357=ORIENTED_EDGE('',*,*,#5855,.F.);
#8358=ORIENTED_EDGE('',*,*,#5840,.T.);
#8359=ORIENTED_EDGE('',*,*,#5856,.F.);
#8360=ORIENTED_EDGE('',*,*,#5857,.T.);
#8361=ORIENTED_EDGE('',*,*,#5853,.F.);
#8362=ORIENTED_EDGE('',*,*,#5858,.T.);
#8363=ORIENTED_EDGE('',*,*,#5859,.T.);
#8364=ORIENTED_EDGE('',*,*,#5856,.T.);
#8365=ORIENTED_EDGE('',*,*,#5843,.T.);
#8366=ORIENTED_EDGE('',*,*,#5860,.T.);
#8367=ORIENTED_EDGE('',*,*,#5824,.T.);
#8368=ORIENTED_EDGE('',*,*,#5861,.F.);
#8369=ORIENTED_EDGE('',*,*,#5862,.T.);
#8370=ORIENTED_EDGE('',*,*,#5837,.F.);
#8371=ORIENTED_EDGE('',*,*,#5863,.T.);
#8372=ORIENTED_EDGE('',*,*,#5864,.T.);
#8373=ORIENTED_EDGE('',*,*,#5861,.T.);
#8374=ORIENTED_EDGE('',*,*,#5827,.T.);
#8375=ORIENTED_EDGE('',*,*,#5865,.T.);
#8376=ORIENTED_EDGE('',*,*,#5845,.T.);
#8377=ORIENTED_EDGE('',*,*,#5849,.T.);
#8378=ORIENTED_EDGE('',*,*,#5866,.T.);
#8379=ORIENTED_EDGE('',*,*,#5835,.T.);
#8380=ORIENTED_EDGE('',*,*,#5839,.T.);
#8381=ORIENTED_EDGE('',*,*,#5867,.T.);
#8382=ORIENTED_EDGE('',*,*,#5808,.T.);
#8383=ORIENTED_EDGE('',*,*,#5868,.F.);
#8384=ORIENTED_EDGE('',*,*,#5869,.T.);
#8385=ORIENTED_EDGE('',*,*,#5821,.F.);
#8386=ORIENTED_EDGE('',*,*,#5870,.T.);
#8387=ORIENTED_EDGE('',*,*,#5871,.T.);
#8388=ORIENTED_EDGE('',*,*,#5813,.T.);
#8389=ORIENTED_EDGE('',*,*,#5817,.T.);
#8390=ORIENTED_EDGE('',*,*,#5872,.T.);
#8391=ORIENTED_EDGE('',*,*,#5792,.T.);
#8392=ORIENTED_EDGE('',*,*,#5873,.F.);
#8393=ORIENTED_EDGE('',*,*,#5874,.T.);
#8394=ORIENTED_EDGE('',*,*,#5805,.F.);
#8395=ORIENTED_EDGE('',*,*,#5875,.T.);
#8396=ORIENTED_EDGE('',*,*,#5876,.T.);
#8397=ORIENTED_EDGE('',*,*,#5803,.T.);
#8398=ORIENTED_EDGE('',*,*,#5807,.T.);
#8399=ORIENTED_EDGE('',*,*,#5877,.T.);
#8400=ORIENTED_EDGE('',*,*,#5829,.T.);
#8401=ORIENTED_EDGE('',*,*,#5833,.T.);
#8402=ORIENTED_EDGE('',*,*,#5878,.T.);
#8403=ORIENTED_EDGE('',*,*,#5797,.T.);
#8404=ORIENTED_EDGE('',*,*,#5801,.T.);
#8405=ORIENTED_EDGE('',*,*,#5879,.T.);
#8406=ORIENTED_EDGE('',*,*,#5873,.T.);
#8407=ORIENTED_EDGE('',*,*,#5795,.T.);
#8408=ORIENTED_EDGE('',*,*,#5880,.T.);
#8409=ORIENTED_EDGE('',*,*,#5868,.T.);
#8410=ORIENTED_EDGE('',*,*,#5811,.T.);
#8411=ORIENTED_EDGE('',*,*,#5881,.T.);
#8412=ORIENTED_EDGE('',*,*,#5819,.T.);
#8413=ORIENTED_EDGE('',*,*,#5823,.T.);
#8414=ORIENTED_EDGE('',*,*,#5882,.T.);
#8415=ORIENTED_EDGE('',*,*,#5851,.T.);
#8416=ORIENTED_EDGE('',*,*,#5855,.T.);
#8417=ORIENTED_EDGE('',*,*,#5883,.T.);
#8418=ORIENTED_EDGE('',*,*,#5860,.F.);
#8419=ORIENTED_EDGE('',*,*,#5842,.F.);
#8420=ORIENTED_EDGE('',*,*,#5846,.F.);
#8421=ORIENTED_EDGE('',*,*,#5867,.F.);
#8422=ORIENTED_EDGE('',*,*,#5838,.F.);
#8423=ORIENTED_EDGE('',*,*,#5862,.F.);
#8424=ORIENTED_EDGE('',*,*,#5864,.F.);
#8425=ORIENTED_EDGE('',*,*,#5884,.F.);
#8426=ORIENTED_EDGE('',*,*,#5885,.T.);
#8427=ORIENTED_EDGE('',*,*,#5886,.T.);
#8428=ORIENTED_EDGE('',*,*,#5887,.T.);
#8429=ORIENTED_EDGE('',*,*,#5888,.F.);
#8430=ORIENTED_EDGE('',*,*,#5889,.F.);
#8431=ORIENTED_EDGE('',*,*,#5890,.T.);
#8432=ORIENTED_EDGE('',*,*,#5891,.T.);
#8433=ORIENTED_EDGE('',*,*,#5892,.T.);
#8434=ORIENTED_EDGE('',*,*,#5863,.F.);
#8435=ORIENTED_EDGE('',*,*,#5893,.F.);
#8436=ORIENTED_EDGE('',*,*,#5894,.T.);
#8437=ORIENTED_EDGE('',*,*,#5895,.F.);
#8438=ORIENTED_EDGE('',*,*,#5896,.T.);
#8439=ORIENTED_EDGE('',*,*,#5897,.T.);
#8440=ORIENTED_EDGE('',*,*,#5884,.T.);
#8441=ORIENTED_EDGE('',*,*,#5865,.F.);
#8442=ORIENTED_EDGE('',*,*,#5826,.F.);
#8443=ORIENTED_EDGE('',*,*,#5830,.F.);
#8444=ORIENTED_EDGE('',*,*,#5879,.F.);
#8445=ORIENTED_EDGE('',*,*,#5800,.F.);
#8446=ORIENTED_EDGE('',*,*,#5804,.F.);
#8447=ORIENTED_EDGE('',*,*,#5876,.F.);
#8448=ORIENTED_EDGE('',*,*,#5898,.T.);
#8449=ORIENTED_EDGE('',*,*,#5899,.T.);
#8450=ORIENTED_EDGE('',*,*,#5900,.F.);
#8451=ORIENTED_EDGE('',*,*,#5901,.F.);
#8452=ORIENTED_EDGE('',*,*,#5902,.T.);
#8453=ORIENTED_EDGE('',*,*,#5903,.T.);
#8454=ORIENTED_EDGE('',*,*,#5904,.F.);
#8455=ORIENTED_EDGE('',*,*,#5905,.F.);
#8456=ORIENTED_EDGE('',*,*,#5893,.T.);
#8457=ORIENTED_EDGE('',*,*,#5875,.F.);
#8458=ORIENTED_EDGE('',*,*,#5906,.F.);
#8459=ORIENTED_EDGE('',*,*,#5907,.F.);
#8460=ORIENTED_EDGE('',*,*,#5908,.F.);
#8461=ORIENTED_EDGE('',*,*,#5909,.F.);
#8462=ORIENTED_EDGE('',*,*,#5910,.T.);
#8463=ORIENTED_EDGE('',*,*,#5898,.F.);
#8464=ORIENTED_EDGE('',*,*,#5798,.F.);
#8465=ORIENTED_EDGE('',*,*,#5878,.F.);
#8466=ORIENTED_EDGE('',*,*,#5832,.F.);
#8467=ORIENTED_EDGE('',*,*,#5836,.F.);
#8468=ORIENTED_EDGE('',*,*,#5866,.F.);
#8469=ORIENTED_EDGE('',*,*,#5848,.F.);
#8470=ORIENTED_EDGE('',*,*,#5852,.F.);
#8471=ORIENTED_EDGE('',*,*,#5882,.F.);
#8472=ORIENTED_EDGE('',*,*,#5822,.F.);
#8473=ORIENTED_EDGE('',*,*,#5869,.F.);
#8474=ORIENTED_EDGE('',*,*,#5880,.F.);
#8475=ORIENTED_EDGE('',*,*,#5794,.F.);
#8476=ORIENTED_EDGE('',*,*,#5911,.F.);
#8477=ORIENTED_EDGE('',*,*,#5912,.T.);
#8478=ORIENTED_EDGE('',*,*,#5913,.T.);
#8479=ORIENTED_EDGE('',*,*,#5914,.T.);
#8480=ORIENTED_EDGE('',*,*,#5915,.T.);
#8481=ORIENTED_EDGE('',*,*,#5916,.T.);
#8482=ORIENTED_EDGE('',*,*,#5914,.F.);
#8483=ORIENTED_EDGE('',*,*,#5917,.T.);
#8484=ORIENTED_EDGE('',*,*,#5900,.T.);
#8485=ORIENTED_EDGE('',*,*,#5918,.T.);
#8486=ORIENTED_EDGE('',*,*,#5913,.F.);
#8487=ORIENTED_EDGE('',*,*,#5919,.F.);
#8488=ORIENTED_EDGE('',*,*,#5920,.T.);
#8489=ORIENTED_EDGE('',*,*,#5921,.F.);
#8490=ORIENTED_EDGE('',*,*,#5901,.T.);
#8491=ORIENTED_EDGE('',*,*,#5917,.F.);
#8492=ORIENTED_EDGE('',*,*,#5922,.T.);
#8493=ORIENTED_EDGE('',*,*,#5923,.T.);
#8494=ORIENTED_EDGE('',*,*,#5924,.T.);
#8495=ORIENTED_EDGE('',*,*,#5925,.T.);
#8496=ORIENTED_EDGE('',*,*,#5923,.F.);
#8497=ORIENTED_EDGE('',*,*,#5926,.T.);
#8498=ORIENTED_EDGE('',*,*,#5904,.T.);
#8499=ORIENTED_EDGE('',*,*,#5927,.T.);
#8500=ORIENTED_EDGE('',*,*,#5922,.F.);
#8501=ORIENTED_EDGE('',*,*,#5928,.F.);
#8502=ORIENTED_EDGE('',*,*,#5929,.F.);
#8503=ORIENTED_EDGE('',*,*,#5894,.F.);
#8504=ORIENTED_EDGE('',*,*,#5905,.T.);
#8505=ORIENTED_EDGE('',*,*,#5926,.F.);
#8506=ORIENTED_EDGE('',*,*,#5930,.T.);
#8507=ORIENTED_EDGE('',*,*,#5931,.T.);
#8508=ORIENTED_EDGE('',*,*,#5932,.T.);
#8509=ORIENTED_EDGE('',*,*,#5933,.T.);
#8510=ORIENTED_EDGE('',*,*,#5932,.F.);
#8511=ORIENTED_EDGE('',*,*,#5934,.F.);
#8512=ORIENTED_EDGE('',*,*,#5887,.F.);
#8513=ORIENTED_EDGE('',*,*,#5935,.F.);
#8514=ORIENTED_EDGE('',*,*,#5936,.T.);
#8515=ORIENTED_EDGE('',*,*,#5937,.T.);
#8516=ORIENTED_EDGE('',*,*,#5938,.T.);
#8517=ORIENTED_EDGE('',*,*,#5931,.F.);
#8518=ORIENTED_EDGE('',*,*,#5939,.T.);
#8519=ORIENTED_EDGE('',*,*,#5888,.T.);
#8520=ORIENTED_EDGE('',*,*,#5934,.T.);
#8521=ORIENTED_EDGE('',*,*,#5940,.T.);
#8522=ORIENTED_EDGE('',*,*,#5941,.T.);
#8523=ORIENTED_EDGE('',*,*,#5942,.T.);
#8524=ORIENTED_EDGE('',*,*,#5943,.T.);
#8525=ORIENTED_EDGE('',*,*,#5942,.F.);
#8526=ORIENTED_EDGE('',*,*,#5944,.F.);
#8527=ORIENTED_EDGE('',*,*,#5945,.F.);
#8528=ORIENTED_EDGE('',*,*,#5946,.F.);
#8529=ORIENTED_EDGE('',*,*,#5947,.T.);
#8530=ORIENTED_EDGE('',*,*,#5948,.F.);
#8531=ORIENTED_EDGE('',*,*,#5949,.T.);
#8532=ORIENTED_EDGE('',*,*,#5941,.F.);
#8533=ORIENTED_EDGE('',*,*,#5950,.T.);
#8534=ORIENTED_EDGE('',*,*,#5951,.T.);
#8535=ORIENTED_EDGE('',*,*,#5944,.T.);
#8536=ORIENTED_EDGE('',*,*,#5952,.T.);
#8537=ORIENTED_EDGE('',*,*,#5953,.T.);
#8538=ORIENTED_EDGE('',*,*,#5954,.T.);
#8539=ORIENTED_EDGE('',*,*,#5955,.T.);
#8540=ORIENTED_EDGE('',*,*,#5953,.F.);
#8541=ORIENTED_EDGE('',*,*,#5956,.T.);
#8542=ORIENTED_EDGE('',*,*,#5957,.T.);
#8543=ORIENTED_EDGE('',*,*,#5958,.T.);
#8544=ORIENTED_EDGE('',*,*,#5952,.F.);
#8545=ORIENTED_EDGE('',*,*,#5959,.F.);
#8546=ORIENTED_EDGE('',*,*,#5960,.F.);
#8547=ORIENTED_EDGE('',*,*,#5961,.F.);
#8548=ORIENTED_EDGE('',*,*,#5962,.T.);
#8549=ORIENTED_EDGE('',*,*,#5956,.F.);
#8550=ORIENTED_EDGE('',*,*,#5963,.F.);
#8551=ORIENTED_EDGE('',*,*,#5960,.T.);
#8552=ORIENTED_EDGE('',*,*,#5964,.T.);
#8553=ORIENTED_EDGE('',*,*,#5965,.T.);
#8554=ORIENTED_EDGE('',*,*,#5955,.F.);
#8555=ORIENTED_EDGE('',*,*,#5966,.F.);
#8556=ORIENTED_EDGE('',*,*,#5964,.F.);
#8557=ORIENTED_EDGE('',*,*,#5959,.T.);
#8558=ORIENTED_EDGE('',*,*,#5954,.F.);
#8559=ORIENTED_EDGE('',*,*,#5958,.F.);
#8560=ORIENTED_EDGE('',*,*,#5967,.F.);
#8561=ORIENTED_EDGE('',*,*,#5968,.F.);
#8562=ORIENTED_EDGE('',*,*,#5965,.F.);
#8563=ORIENTED_EDGE('',*,*,#5966,.T.);
#8564=ORIENTED_EDGE('',*,*,#5870,.F.);
#8565=ORIENTED_EDGE('',*,*,#5969,.F.);
#8566=ORIENTED_EDGE('',*,*,#5961,.T.);
#8567=ORIENTED_EDGE('',*,*,#5970,.F.);
#8568=ORIENTED_EDGE('',*,*,#5971,.F.);
#8569=ORIENTED_EDGE('',*,*,#5972,.T.);
#8570=ORIENTED_EDGE('',*,*,#5973,.T.);
#8571=ORIENTED_EDGE('',*,*,#5858,.F.);
#8572=ORIENTED_EDGE('',*,*,#5892,.F.);
#8573=ORIENTED_EDGE('',*,*,#5974,.F.);
#8574=ORIENTED_EDGE('',*,*,#5975,.T.);
#8575=ORIENTED_EDGE('',*,*,#5976,.F.);
#8576=ORIENTED_EDGE('',*,*,#5968,.T.);
#8577=ORIENTED_EDGE('',*,*,#5977,.F.);
#8578=ORIENTED_EDGE('',*,*,#5916,.F.);
#8579=ORIENTED_EDGE('',*,*,#5978,.F.);
#8580=ORIENTED_EDGE('',*,*,#5979,.T.);
#8581=ORIENTED_EDGE('',*,*,#5919,.T.);
#8582=ORIENTED_EDGE('',*,*,#5915,.F.);
#8583=ORIENTED_EDGE('',*,*,#5918,.F.);
#8584=ORIENTED_EDGE('',*,*,#5899,.F.);
#8585=ORIENTED_EDGE('',*,*,#5910,.F.);
#8586=ORIENTED_EDGE('',*,*,#5980,.T.);
#8587=ORIENTED_EDGE('',*,*,#5978,.T.);
#8588=ORIENTED_EDGE('',*,*,#5981,.F.);
#8589=ORIENTED_EDGE('',*,*,#5920,.F.);
#8590=ORIENTED_EDGE('',*,*,#5979,.F.);
#8591=ORIENTED_EDGE('',*,*,#5980,.F.);
#8592=ORIENTED_EDGE('',*,*,#5921,.T.);
#8593=ORIENTED_EDGE('',*,*,#5982,.F.);
#8594=ORIENTED_EDGE('',*,*,#5983,.T.);
#8595=ORIENTED_EDGE('',*,*,#5902,.F.);
#8596=ORIENTED_EDGE('',*,*,#5943,.F.);
#8597=ORIENTED_EDGE('',*,*,#5949,.F.);
#8598=ORIENTED_EDGE('',*,*,#5984,.F.);
#8599=ORIENTED_EDGE('',*,*,#5985,.T.);
#8600=ORIENTED_EDGE('',*,*,#5986,.F.);
#8601=ORIENTED_EDGE('',*,*,#5987,.T.);
#8602=ORIENTED_EDGE('',*,*,#5984,.T.);
#8603=ORIENTED_EDGE('',*,*,#5948,.T.);
#8604=ORIENTED_EDGE('',*,*,#5988,.F.);
#8605=ORIENTED_EDGE('',*,*,#5929,.T.);
#8606=ORIENTED_EDGE('',*,*,#5989,.T.);
#8607=ORIENTED_EDGE('',*,*,#5990,.T.);
#8608=ORIENTED_EDGE('',*,*,#5925,.F.);
#8609=ORIENTED_EDGE('',*,*,#5991,.F.);
#8610=ORIENTED_EDGE('',*,*,#5989,.F.);
#8611=ORIENTED_EDGE('',*,*,#5928,.T.);
#8612=ORIENTED_EDGE('',*,*,#5924,.F.);
#8613=ORIENTED_EDGE('',*,*,#5927,.F.);
#8614=ORIENTED_EDGE('',*,*,#5903,.F.);
#8615=ORIENTED_EDGE('',*,*,#5983,.F.);
#8616=ORIENTED_EDGE('',*,*,#5990,.F.);
#8617=ORIENTED_EDGE('',*,*,#5991,.T.);
#8618=ORIENTED_EDGE('',*,*,#5933,.F.);
#8619=ORIENTED_EDGE('',*,*,#5938,.F.);
#8620=ORIENTED_EDGE('',*,*,#5992,.T.);
#8621=ORIENTED_EDGE('',*,*,#5993,.T.);
#8622=ORIENTED_EDGE('',*,*,#5994,.T.);
#8623=ORIENTED_EDGE('',*,*,#5995,.F.);
#8624=ORIENTED_EDGE('',*,*,#5992,.F.);
#8625=ORIENTED_EDGE('',*,*,#5937,.F.);
#8626=ORIENTED_EDGE('',*,*,#5911,.T.);
#8627=ORIENTED_EDGE('',*,*,#5996,.T.);
#8628=ORIENTED_EDGE('',*,*,#5997,.F.);
#8629=ORIENTED_EDGE('',*,*,#5996,.F.);
#8630=ORIENTED_EDGE('',*,*,#5998,.F.);
#8631=ORIENTED_EDGE('',*,*,#5999,.T.);
#8632=ORIENTED_EDGE('',*,*,#6000,.F.);
#8633=ORIENTED_EDGE('',*,*,#5999,.F.);
#8634=ORIENTED_EDGE('',*,*,#5997,.T.);
#8635=ORIENTED_EDGE('',*,*,#6000,.T.);
#8636=ORIENTED_EDGE('',*,*,#6001,.T.);
#8637=ORIENTED_EDGE('',*,*,#6002,.F.);
#8638=ORIENTED_EDGE('',*,*,#6003,.F.);
#8639=ORIENTED_EDGE('',*,*,#6004,.F.);
#8640=ORIENTED_EDGE('',*,*,#6005,.T.);
#8641=ORIENTED_EDGE('',*,*,#6006,.F.);
#8642=ORIENTED_EDGE('',*,*,#5998,.T.);
#8643=ORIENTED_EDGE('',*,*,#6001,.F.);
#8644=ORIENTED_EDGE('',*,*,#6007,.T.);
#8645=ORIENTED_EDGE('',*,*,#5912,.F.);
#8646=ORIENTED_EDGE('',*,*,#6007,.F.);
#8647=ORIENTED_EDGE('',*,*,#6008,.F.);
#8648=ORIENTED_EDGE('',*,*,#5970,.T.);
#8649=ORIENTED_EDGE('',*,*,#5963,.T.);
#8650=ORIENTED_EDGE('',*,*,#5976,.T.);
#8651=ORIENTED_EDGE('',*,*,#6009,.T.);
#8652=ORIENTED_EDGE('',*,*,#6004,.T.);
#8653=ORIENTED_EDGE('',*,*,#5859,.F.);
#8654=ORIENTED_EDGE('',*,*,#5977,.T.);
#8655=ORIENTED_EDGE('',*,*,#5967,.T.);
#8656=ORIENTED_EDGE('',*,*,#5957,.F.);
#8657=ORIENTED_EDGE('',*,*,#5962,.F.);
#8658=ORIENTED_EDGE('',*,*,#5969,.T.);
#8659=ORIENTED_EDGE('',*,*,#5872,.F.);
#8660=ORIENTED_EDGE('',*,*,#5816,.F.);
#8661=ORIENTED_EDGE('',*,*,#5820,.F.);
#8662=ORIENTED_EDGE('',*,*,#5883,.F.);
#8663=ORIENTED_EDGE('',*,*,#5854,.F.);
#8664=ORIENTED_EDGE('',*,*,#5857,.F.);
#8665=ORIENTED_EDGE('',*,*,#6010,.F.);
#8666=ORIENTED_EDGE('',*,*,#5994,.F.);
#8667=ORIENTED_EDGE('',*,*,#5936,.F.);
#8668=ORIENTED_EDGE('',*,*,#6011,.F.);
#8669=ORIENTED_EDGE('',*,*,#6012,.F.);
#8670=ORIENTED_EDGE('',*,*,#5896,.F.);
#8671=ORIENTED_EDGE('',*,*,#6013,.F.);
#8672=ORIENTED_EDGE('',*,*,#6005,.F.);
#8673=ORIENTED_EDGE('',*,*,#6009,.F.);
#8674=ORIENTED_EDGE('',*,*,#5975,.F.);
#8675=ORIENTED_EDGE('',*,*,#6014,.F.);
#8676=ORIENTED_EDGE('',*,*,#6015,.F.);
#8677=ORIENTED_EDGE('',*,*,#6012,.T.);
#8678=ORIENTED_EDGE('',*,*,#6016,.T.);
#8679=ORIENTED_EDGE('',*,*,#5885,.F.);
#8680=ORIENTED_EDGE('',*,*,#5897,.F.);
#8681=ORIENTED_EDGE('',*,*,#6011,.T.);
#8682=ORIENTED_EDGE('',*,*,#5935,.T.);
#8683=ORIENTED_EDGE('',*,*,#5886,.F.);
#8684=ORIENTED_EDGE('',*,*,#6016,.F.);
#8685=ORIENTED_EDGE('',*,*,#5930,.F.);
#8686=ORIENTED_EDGE('',*,*,#5993,.F.);
#8687=ORIENTED_EDGE('',*,*,#5995,.T.);
#8688=ORIENTED_EDGE('',*,*,#6010,.T.);
#8689=ORIENTED_EDGE('',*,*,#6017,.T.);
#8690=ORIENTED_EDGE('',*,*,#5889,.T.);
#8691=ORIENTED_EDGE('',*,*,#5939,.F.);
#8692=ORIENTED_EDGE('',*,*,#6014,.T.);
#8693=ORIENTED_EDGE('',*,*,#5974,.T.);
#8694=ORIENTED_EDGE('',*,*,#5891,.F.);
#8695=ORIENTED_EDGE('',*,*,#6018,.F.);
#8696=ORIENTED_EDGE('',*,*,#6015,.T.);
#8697=ORIENTED_EDGE('',*,*,#6018,.T.);
#8698=ORIENTED_EDGE('',*,*,#5890,.F.);
#8699=ORIENTED_EDGE('',*,*,#6017,.F.);
#8700=ORIENTED_EDGE('',*,*,#6013,.T.);
#8701=ORIENTED_EDGE('',*,*,#5895,.T.);
#8702=ORIENTED_EDGE('',*,*,#5988,.T.);
#8703=ORIENTED_EDGE('',*,*,#5982,.T.);
#8704=ORIENTED_EDGE('',*,*,#5981,.T.);
#8705=ORIENTED_EDGE('',*,*,#5909,.T.);
#8706=ORIENTED_EDGE('',*,*,#6019,.F.);
#8707=ORIENTED_EDGE('',*,*,#6002,.T.);
#8708=ORIENTED_EDGE('',*,*,#6006,.T.);
#8709=ORIENTED_EDGE('',*,*,#6020,.F.);
#8710=ORIENTED_EDGE('',*,*,#5946,.T.);
#8711=ORIENTED_EDGE('',*,*,#6021,.F.);
#8712=ORIENTED_EDGE('',*,*,#6022,.F.);
#8713=ORIENTED_EDGE('',*,*,#6023,.F.);
#8714=ORIENTED_EDGE('',*,*,#6022,.T.);
#8715=ORIENTED_EDGE('',*,*,#6024,.F.);
#8716=ORIENTED_EDGE('',*,*,#5972,.F.);
#8717=ORIENTED_EDGE('',*,*,#6025,.T.);
#8718=ORIENTED_EDGE('',*,*,#5907,.T.);
#8719=ORIENTED_EDGE('',*,*,#6026,.F.);
#8720=ORIENTED_EDGE('',*,*,#6027,.F.);
#8721=ORIENTED_EDGE('',*,*,#6028,.F.);
#8722=ORIENTED_EDGE('',*,*,#6027,.T.);
#8723=ORIENTED_EDGE('',*,*,#6029,.F.);
#8724=ORIENTED_EDGE('',*,*,#6030,.F.);
#8725=ORIENTED_EDGE('',*,*,#5940,.F.);
#8726=ORIENTED_EDGE('',*,*,#5985,.F.);
#8727=ORIENTED_EDGE('',*,*,#5987,.F.);
#8728=ORIENTED_EDGE('',*,*,#6031,.F.);
#8729=ORIENTED_EDGE('',*,*,#6030,.T.);
#8730=ORIENTED_EDGE('',*,*,#6032,.T.);
#8731=ORIENTED_EDGE('',*,*,#5950,.F.);
#8732=ORIENTED_EDGE('',*,*,#5871,.F.);
#8733=ORIENTED_EDGE('',*,*,#5973,.F.);
#8734=ORIENTED_EDGE('',*,*,#6024,.T.);
#8735=ORIENTED_EDGE('',*,*,#6021,.T.);
#8736=ORIENTED_EDGE('',*,*,#5945,.T.);
#8737=ORIENTED_EDGE('',*,*,#5951,.F.);
#8738=ORIENTED_EDGE('',*,*,#6032,.F.);
#8739=ORIENTED_EDGE('',*,*,#6029,.T.);
#8740=ORIENTED_EDGE('',*,*,#6026,.T.);
#8741=ORIENTED_EDGE('',*,*,#5906,.T.);
#8742=ORIENTED_EDGE('',*,*,#5877,.F.);
#8743=ORIENTED_EDGE('',*,*,#5806,.F.);
#8744=ORIENTED_EDGE('',*,*,#5874,.F.);
#8745=ORIENTED_EDGE('',*,*,#5881,.F.);
#8746=ORIENTED_EDGE('',*,*,#5810,.F.);
#8747=ORIENTED_EDGE('',*,*,#5814,.F.);
#8748=ORIENTED_EDGE('',*,*,#5947,.F.);
#8749=ORIENTED_EDGE('',*,*,#6020,.T.);
#8750=ORIENTED_EDGE('',*,*,#6023,.T.);
#8751=ORIENTED_EDGE('',*,*,#5971,.T.);
#8752=ORIENTED_EDGE('',*,*,#6008,.T.);
#8753=ORIENTED_EDGE('',*,*,#6003,.T.);
#8754=ORIENTED_EDGE('',*,*,#6019,.T.);
#8755=ORIENTED_EDGE('',*,*,#5908,.T.);
#8756=ORIENTED_EDGE('',*,*,#6025,.F.);
#8757=ORIENTED_EDGE('',*,*,#6028,.T.);
#8758=ORIENTED_EDGE('',*,*,#6031,.T.);
#8759=ORIENTED_EDGE('',*,*,#5986,.T.);
#9261=CYLINDRICAL_SURFACE('',#10791,0.00075);
#9262=CYLINDRICAL_SURFACE('',#10795,0.00075);
#9263=CYLINDRICAL_SURFACE('',#10797,0.00075);
#9264=CYLINDRICAL_SURFACE('',#10800,0.00075);
#9265=CYLINDRICAL_SURFACE('',#10804,0.00075);
#9266=CYLINDRICAL_SURFACE('',#10806,0.00075);
#9267=CYLINDRICAL_SURFACE('',#10807,0.00075);
#9268=CYLINDRICAL_SURFACE('',#10808,0.00075);
#9269=CYLINDRICAL_SURFACE('',#10818,0.001);
#9270=CYLINDRICAL_SURFACE('',#10823,0.001);
#9271=CYLINDRICAL_SURFACE('',#10828,0.001);
#9272=CYLINDRICAL_SURFACE('',#10833,0.001);
#9273=CYLINDRICAL_SURFACE('',#10838,0.001);
#9274=CYLINDRICAL_SURFACE('',#10862,0.0041);
#9275=CYLINDRICAL_SURFACE('',#10868,0.0025);
#9276=CYLINDRICAL_SURFACE('',#10875,0.003);
#9277=CYLINDRICAL_SURFACE('',#10878,0.00155);
#9278=CYLINDRICAL_SURFACE('',#10880,0.00155);
#9279=CYLINDRICAL_SURFACE('',#10885,0.003);
#9695=ADVANCED_FACE('',(#1473),#115,.T.);
#9696=ADVANCED_FACE('',(#1474),#116,.T.);
#9697=ADVANCED_FACE('',(#1475),#117,.T.);
#9698=ADVANCED_FACE('',(#1476),#118,.T.);
#9699=ADVANCED_FACE('',(#1477),#119,.T.);
#9700=ADVANCED_FACE('',(#1478),#120,.T.);
#9701=ADVANCED_FACE('',(#1479),#121,.T.);
#9702=ADVANCED_FACE('',(#1480),#122,.T.);
#9703=ADVANCED_FACE('',(#1481),#123,.T.);
#9704=ADVANCED_FACE('',(#1482),#124,.T.);
#9705=ADVANCED_FACE('',(#1483),#125,.T.);
#9706=ADVANCED_FACE('',(#1484),#126,.T.);
#9707=ADVANCED_FACE('',(#1485),#127,.T.);
#9708=ADVANCED_FACE('',(#1486),#128,.T.);
#9709=ADVANCED_FACE('',(#1487),#129,.T.);
#9710=ADVANCED_FACE('',(#1488),#130,.T.);
#9711=ADVANCED_FACE('',(#1489),#131,.T.);
#9712=ADVANCED_FACE('',(#1490),#132,.T.);
#9713=ADVANCED_FACE('',(#1491),#133,.T.);
#9714=ADVANCED_FACE('',(#1492),#134,.T.);
#9715=ADVANCED_FACE('',(#1493),#135,.T.);
#9716=ADVANCED_FACE('',(#1494),#9261,.T.);
#9717=ADVANCED_FACE('',(#1495),#136,.T.);
#9718=ADVANCED_FACE('',(#1496),#9262,.T.);
#9719=ADVANCED_FACE('',(#1497),#9263,.T.);
#9720=ADVANCED_FACE('',(#1498),#137,.T.);
#9721=ADVANCED_FACE('',(#1499),#9264,.T.);
#9722=ADVANCED_FACE('',(#1500),#138,.T.);
#9723=ADVANCED_FACE('',(#1501),#9265,.T.);
#9724=ADVANCED_FACE('',(#1502),#9266,.T.);
#9725=ADVANCED_FACE('',(#1503),#9267,.T.);
#9726=ADVANCED_FACE('',(#1504),#9268,.T.);
#9727=ADVANCED_FACE('',(#1505),#1038,.T.);
#9728=ADVANCED_FACE('',(#1506),#1039,.T.);
#9729=ADVANCED_FACE('',(#1507),#1040,.T.);
#9730=ADVANCED_FACE('',(#1508),#1041,.T.);
#9731=ADVANCED_FACE('',(#1509,#760,#761),#1042,.F.);
#9732=ADVANCED_FACE('',(#1510),#9269,.T.);
#9733=ADVANCED_FACE('',(#1511),#1043,.T.);
#9734=ADVANCED_FACE('',(#1512),#1044,.T.);
#9735=ADVANCED_FACE('',(#1513),#9270,.T.);
#9736=ADVANCED_FACE('',(#1514),#1045,.T.);
#9737=ADVANCED_FACE('',(#1515),#1046,.T.);
#9738=ADVANCED_FACE('',(#1516),#9271,.T.);
#9739=ADVANCED_FACE('',(#1517),#1047,.T.);
#9740=ADVANCED_FACE('',(#1518),#1048,.T.);
#9741=ADVANCED_FACE('',(#1519),#9272,.T.);
#9742=ADVANCED_FACE('',(#1520),#1049,.T.);
#9743=ADVANCED_FACE('',(#1521),#1050,.T.);
#9744=ADVANCED_FACE('',(#1522),#9273,.T.);
#9745=ADVANCED_FACE('',(#1523),#1051,.T.);
#9746=ADVANCED_FACE('',(#1524),#1052,.T.);
#9747=ADVANCED_FACE('',(#1525),#1053,.F.);
#9748=ADVANCED_FACE('',(#1526),#1054,.T.);
#9749=ADVANCED_FACE('',(#1527),#1055,.T.);
#9750=ADVANCED_FACE('',(#1528),#1056,.T.);
#9751=ADVANCED_FACE('',(#1529),#1057,.T.);
#9752=ADVANCED_FACE('',(#1530),#1058,.T.);
#9753=ADVANCED_FACE('',(#1531),#1059,.T.);
#9754=ADVANCED_FACE('',(#1532),#1060,.F.);
#9755=ADVANCED_FACE('',(#1533),#1061,.T.);
#9756=ADVANCED_FACE('',(#1534),#1062,.T.);
#9757=ADVANCED_FACE('',(#1535),#1063,.F.);
#9758=ADVANCED_FACE('',(#1536),#1064,.F.);
#9759=ADVANCED_FACE('',(#1537),#1065,.T.);
#9760=ADVANCED_FACE('',(#1538),#1066,.T.);
#9761=ADVANCED_FACE('',(#1539),#1067,.T.);
#9762=ADVANCED_FACE('',(#1540),#1068,.F.);
#9763=ADVANCED_FACE('',(#1541),#777,.F.);
#9764=ADVANCED_FACE('',(#1542),#9274,.F.);
#9765=ADVANCED_FACE('',(#1543,#762),#1069,.T.);
#9766=ADVANCED_FACE('',(#1544,#763),#1070,.T.);
#9767=ADVANCED_FACE('',(#1545),#9275,.F.);
#9768=ADVANCED_FACE('',(#1546),#1071,.F.);
#9769=ADVANCED_FACE('',(#1547),#1072,.T.);
#9770=ADVANCED_FACE('',(#1548),#1073,.T.);
#9771=ADVANCED_FACE('',(#1549),#1074,.T.);
#9772=ADVANCED_FACE('',(#1550),#9276,.F.);
#9773=ADVANCED_FACE('',(#1551),#1075,.T.);
#9774=ADVANCED_FACE('',(#1552),#1076,.T.);
#9775=ADVANCED_FACE('',(#1553),#9277,.F.);
#9776=ADVANCED_FACE('',(#1554),#1077,.F.);
#9777=ADVANCED_FACE('',(#1555),#9278,.F.);
#9778=ADVANCED_FACE('',(#1556),#1078,.T.);
#9779=ADVANCED_FACE('',(#1557),#1079,.T.);
#9780=ADVANCED_FACE('',(#1558),#9279,.F.);
#9781=ADVANCED_FACE('',(#1559),#1080,.T.);
#9782=ADVANCED_FACE('',(#1560),#1081,.T.);
#9783=ADVANCED_FACE('',(#1561),#1082,.F.);
#9879=CLOSED_SHELL('',(#9695,#9696,#9697,#9698,#9699,#9700,#9701,#9702,
#9703,#9704,#9705,#9706,#9707,#9708,#9709,#9710,#9711,#9712,#9713,#9714,
#9715,#9716,#9717,#9718,#9719,#9720,#9721,#9722,#9723,#9724,#9725,#9726,
#9727,#9728,#9729,#9730,#9731,#9732,#9733,#9734,#9735,#9736,#9737,#9738,
#9739,#9740,#9741,#9742,#9743,#9744,#9745,#9746,#9747,#9748,#9749,#9750,
#9751,#9752,#9753,#9754,#9755,#9756,#9757,#9758,#9759,#9760,#9761,#9762,
#9763,#9764,#9765,#9766,#9767,#9768,#9769,#9770,#9771,#9772,#9773,#9774,
#9775,#9776,#9777,#9778,#9779,#9780,#9781,#9782,#9783));
#10748=AXIS2_PLACEMENT_3D('',#44427,#12700,#12701);
#10749=AXIS2_PLACEMENT_3D('',#44480,#12702,#12703);
#10750=AXIS2_PLACEMENT_3D('',#44481,#12704,#12705);
#10751=AXIS2_PLACEMENT_3D('',#44526,#12706,#12707);
#10752=AXIS2_PLACEMENT_3D('',#44527,#12708,#12709);
#10753=AXIS2_PLACEMENT_3D('',#44572,#12710,#12711);
#10754=AXIS2_PLACEMENT_3D('',#44573,#12712,#12713);
#10755=AXIS2_PLACEMENT_3D('',#44618,#12714,#12715);
#10756=AXIS2_PLACEMENT_3D('',#44619,#12716,#12717);
#10757=AXIS2_PLACEMENT_3D('',#44664,#12718,#12719);
#10758=AXIS2_PLACEMENT_3D('',#44665,#12720,#12721);
#10759=AXIS2_PLACEMENT_3D('',#44718,#12722,#12723);
#10760=AXIS2_PLACEMENT_3D('',#44719,#12724,#12725);
#10761=AXIS2_PLACEMENT_3D('',#44764,#12726,#12727);
#10762=AXIS2_PLACEMENT_3D('',#44765,#12728,#12729);
#10763=AXIS2_PLACEMENT_3D('',#44810,#12730,#12731);
#10764=AXIS2_PLACEMENT_3D('',#44811,#12732,#12733);
#10765=AXIS2_PLACEMENT_3D('',#44856,#12734,#12735);
#10766=AXIS2_PLACEMENT_3D('',#44857,#12736,#12737);
#10767=AXIS2_PLACEMENT_3D('',#44902,#12738,#12739);
#10768=AXIS2_PLACEMENT_3D('',#44903,#12740,#12741);
#10769=AXIS2_PLACEMENT_3D('',#44956,#12742,#12743);
#10770=AXIS2_PLACEMENT_3D('',#44957,#12744,#12745);
#10771=AXIS2_PLACEMENT_3D('',#45002,#12746,#12747);
#10772=AXIS2_PLACEMENT_3D('',#45003,#12748,#12749);
#10773=AXIS2_PLACEMENT_3D('',#45048,#12750,#12751);
#10774=AXIS2_PLACEMENT_3D('',#45049,#12752,#12753);
#10775=AXIS2_PLACEMENT_3D('',#45094,#12754,#12755);
#10776=AXIS2_PLACEMENT_3D('',#45095,#12756,#12757);
#10777=AXIS2_PLACEMENT_3D('',#45140,#12758,#12759);
#10778=AXIS2_PLACEMENT_3D('',#45141,#12760,#12761);
#10779=AXIS2_PLACEMENT_3D('',#45194,#12762,#12763);
#10780=AXIS2_PLACEMENT_3D('',#45195,#12764,#12765);
#10781=AXIS2_PLACEMENT_3D('',#45240,#12766,#12767);
#10782=AXIS2_PLACEMENT_3D('',#45241,#12768,#12769);
#10783=AXIS2_PLACEMENT_3D('',#45286,#12770,#12771);
#10784=AXIS2_PLACEMENT_3D('',#45287,#12772,#12773);
#10785=AXIS2_PLACEMENT_3D('',#45332,#12774,#12775);
#10786=AXIS2_PLACEMENT_3D('',#45333,#12776,#12777);
#10787=AXIS2_PLACEMENT_3D('',#45378,#12778,#12779);
#10788=AXIS2_PLACEMENT_3D('',#45379,#12780,#12781);
#10789=AXIS2_PLACEMENT_3D('',#45417,#12782,#12783);
#10790=AXIS2_PLACEMENT_3D('',#45418,#12784,#12785);
#10791=AXIS2_PLACEMENT_3D('',#45419,#12786,#12787);
#10792=AXIS2_PLACEMENT_3D('',#45422,#12788,#12789);
#10793=AXIS2_PLACEMENT_3D('',#45462,#12792,#12793);
#10794=AXIS2_PLACEMENT_3D('',#45463,#12794,#12795);
#10795=AXIS2_PLACEMENT_3D('',#45464,#12796,#12797);
#10796=AXIS2_PLACEMENT_3D('',#45467,#12798,#12799);
#10797=AXIS2_PLACEMENT_3D('',#45470,#12802,#12803);
#10798=AXIS2_PLACEMENT_3D('',#45510,#12806,#12807);
#10799=AXIS2_PLACEMENT_3D('',#45511,#12808,#12809);
#10800=AXIS2_PLACEMENT_3D('',#45512,#12810,#12811);
#10801=AXIS2_PLACEMENT_3D('',#45515,#12812,#12813);
#10802=AXIS2_PLACEMENT_3D('',#45555,#12816,#12817);
#10803=AXIS2_PLACEMENT_3D('',#45556,#12818,#12819);
#10804=AXIS2_PLACEMENT_3D('',#45557,#12820,#12821);
#10805=AXIS2_PLACEMENT_3D('',#45560,#12822,#12823);
#10806=AXIS2_PLACEMENT_3D('',#45563,#12826,#12827);
#10807=AXIS2_PLACEMENT_3D('',#45566,#12830,#12831);
#10808=AXIS2_PLACEMENT_3D('',#45569,#12834,#12835);
#10809=AXIS2_PLACEMENT_3D('',#45572,#12838,#12839);
#10810=AXIS2_PLACEMENT_3D('',#45578,#12842,#12843);
#10811=AXIS2_PLACEMENT_3D('',#45586,#12847,#12848);
#10812=AXIS2_PLACEMENT_3D('',#45590,#12851,#12852);
#10813=AXIS2_PLACEMENT_3D('',#45600,#12858,#12859);
#10814=AXIS2_PLACEMENT_3D('',#45616,#12868,#12869);
#10815=AXIS2_PLACEMENT_3D('',#45626,#12875,#12876);
#10816=AXIS2_PLACEMENT_3D('',#45628,#12877,#12878);
#10817=AXIS2_PLACEMENT_3D('',#45630,#12879,#12880);
#10818=AXIS2_PLACEMENT_3D('',#45631,#12881,#12882);
#10819=AXIS2_PLACEMENT_3D('',#45634,#12883,#12884);
#10820=AXIS2_PLACEMENT_3D('',#45638,#12886,#12887);
#10821=AXIS2_PLACEMENT_3D('',#45640,#12889,#12890);
#10822=AXIS2_PLACEMENT_3D('',#45643,#12893,#12894);
#10823=AXIS2_PLACEMENT_3D('',#45649,#12898,#12899);
#10824=AXIS2_PLACEMENT_3D('',#45652,#12900,#12901);
#10825=AXIS2_PLACEMENT_3D('',#45656,#12903,#12904);
#10826=AXIS2_PLACEMENT_3D('',#45658,#12906,#12907);
#10827=AXIS2_PLACEMENT_3D('',#45661,#12910,#12911);
#10828=AXIS2_PLACEMENT_3D('',#45665,#12914,#12915);
#10829=AXIS2_PLACEMENT_3D('',#45668,#12916,#12917);
#10830=AXIS2_PLACEMENT_3D('',#45672,#12919,#12920);
#10831=AXIS2_PLACEMENT_3D('',#45674,#12922,#12923);
#10832=AXIS2_PLACEMENT_3D('',#45683,#12929,#12930);
#10833=AXIS2_PLACEMENT_3D('',#45685,#12932,#12933);
#10834=AXIS2_PLACEMENT_3D('',#45688,#12934,#12935);
#10835=AXIS2_PLACEMENT_3D('',#45692,#12937,#12938);
#10836=AXIS2_PLACEMENT_3D('',#45694,#12940,#12941);
#10837=AXIS2_PLACEMENT_3D('',#45706,#12948,#12949);
#10838=AXIS2_PLACEMENT_3D('',#45710,#12952,#12953);
#10839=AXIS2_PLACEMENT_3D('',#45713,#12954,#12955);
#10840=AXIS2_PLACEMENT_3D('',#45717,#12957,#12958);
#10841=AXIS2_PLACEMENT_3D('',#45719,#12960,#12961);
#10842=AXIS2_PLACEMENT_3D('',#45725,#12965,#12966);
#10843=AXIS2_PLACEMENT_3D('',#45733,#12971,#12972);
#10844=AXIS2_PLACEMENT_3D('',#45739,#12976,#12977);
#10845=AXIS2_PLACEMENT_3D('',#45741,#12979,#12980);
#10846=AXIS2_PLACEMENT_3D('',#45745,#12983,#12984);
#10847=AXIS2_PLACEMENT_3D('',#45754,#12990,#12991);
#10848=AXIS2_PLACEMENT_3D('',#45761,#12996,#12997);
#10849=AXIS2_PLACEMENT_3D('',#45765,#13000,#13001);
#10850=AXIS2_PLACEMENT_3D('',#45767,#13003,#13004);
#10851=AXIS2_PLACEMENT_3D('',#45769,#13006,#13007);
#10852=AXIS2_PLACEMENT_3D('',#45773,#13010,#13011);
#10853=AXIS2_PLACEMENT_3D('',#45777,#13014,#13015);
#10854=AXIS2_PLACEMENT_3D('',#45781,#13018,#13019);
#10855=AXIS2_PLACEMENT_3D('',#45786,#13023,#13024);
#10856=AXIS2_PLACEMENT_3D('',#45788,#13026,#13027);
#10857=AXIS2_PLACEMENT_3D('',#45789,#13028,#13029);
#10858=AXIS2_PLACEMENT_3D('',#45793,#13032,#13033);
#10859=AXIS2_PLACEMENT_3D('',#45797,#13036,#13037);
#10860=AXIS2_PLACEMENT_3D('',#45799,#13038,#13039);
#10861=AXIS2_PLACEMENT_3D('',#45800,#13040,#13041);
#10862=AXIS2_PLACEMENT_3D('',#45801,#13042,#13043);
#10863=AXIS2_PLACEMENT_3D('',#45803,#13044,#13045);
#10864=AXIS2_PLACEMENT_3D('',#45806,#13047,#13048);
#10865=AXIS2_PLACEMENT_3D('',#45807,#13049,#13050);
#10866=AXIS2_PLACEMENT_3D('',#45808,#13051,#13052);
#10867=AXIS2_PLACEMENT_3D('',#45810,#13053,#13054);
#10868=AXIS2_PLACEMENT_3D('',#45820,#13060,#13061);
#10869=AXIS2_PLACEMENT_3D('',#45822,#13063,#13064);
#10870=AXIS2_PLACEMENT_3D('',#45825,#13067,#13068);
#10871=AXIS2_PLACEMENT_3D('',#45826,#13069,#13070);
#10872=AXIS2_PLACEMENT_3D('',#45830,#13072,#13073);
#10873=AXIS2_PLACEMENT_3D('',#45835,#13077,#13078);
#10874=AXIS2_PLACEMENT_3D('',#45836,#13079,#13080);
#10875=AXIS2_PLACEMENT_3D('',#45838,#13082,#13083);
#10876=AXIS2_PLACEMENT_3D('',#45839,#13084,#13085);
#10877=AXIS2_PLACEMENT_3D('',#45841,#13087,#13088);
#10878=AXIS2_PLACEMENT_3D('',#45843,#13090,#13091);
#10879=AXIS2_PLACEMENT_3D('',#45844,#13092,#13093);
#10880=AXIS2_PLACEMENT_3D('',#45846,#13095,#13096);
#10881=AXIS2_PLACEMENT_3D('',#45848,#13097,#13098);
#10882=AXIS2_PLACEMENT_3D('',#45850,#13099,#13100);
#10883=AXIS2_PLACEMENT_3D('',#45852,#13102,#13103);
#10884=AXIS2_PLACEMENT_3D('',#45855,#13106,#13107);
#10885=AXIS2_PLACEMENT_3D('',#45861,#13111,#13112);
#10886=AXIS2_PLACEMENT_3D('',#45863,#13113,#13114);
#10887=AXIS2_PLACEMENT_3D('',#45865,#13115,#13116);
#10888=AXIS2_PLACEMENT_3D('',#45867,#13118,#13119);
#10889=AXIS2_PLACEMENT_3D('',#45870,#13122,#13123);
#10890=AXIS2_PLACEMENT_3D('',#45871,#13124,#13125);
#12700=DIRECTION('axis',(0.,0.,1.));
#12701=DIRECTION('refdir',(1.,0.,0.));
#12702=DIRECTION('center_axis',(2.22734643137795E-17,1.,1.11022302462516E-15));
#12703=DIRECTION('ref_axis',(-0.707106781186547,-7.69296511685101E-16,0.707106781186548));
#12704=DIRECTION('center_axis',(1.,2.77555756156289E-17,3.04610206107265E-32));
#12705=DIRECTION('ref_axis',(3.53858499469356E-34,-1.11022302462516E-15,
1.));
#12706=DIRECTION('center_axis',(-3.53858499469356E-34,1.11022302462516E-15,
-1.));
#12707=DIRECTION('ref_axis',(-2.22734643137795E-17,-1.,-1.11022302462516E-15));
#12708=DIRECTION('center_axis',(2.22734643137795E-17,1.,1.11022302462516E-15));
#12709=DIRECTION('ref_axis',(-0.707106781186547,-7.69296511685101E-16,0.707106781186548));
#12710=DIRECTION('center_axis',(1.,2.77555756156289E-17,3.04610206107265E-32));
#12711=DIRECTION('ref_axis',(1.96261557335472E-17,-0.707106781186549,0.707106781186546));
#12712=DIRECTION('center_axis',(-3.53858499469356E-34,1.11022302462516E-15,
-1.));
#12713=DIRECTION('ref_axis',(-2.22734643137795E-17,-1.,-1.11022302462516E-15));
#12714=DIRECTION('center_axis',(2.22734643137795E-17,1.,1.11022302462516E-15));
#12715=DIRECTION('ref_axis',(-1.,2.22734643137795E-17,2.50823714187942E-32));
#12716=DIRECTION('center_axis',(1.,2.77555756156289E-17,3.04610206107265E-32));
#12717=DIRECTION('ref_axis',(1.96261557335472E-17,-0.707106781186549,0.707106781186546));
#12718=DIRECTION('center_axis',(-3.53858499469356E-34,1.11022302462516E-15,
-1.));
#12719=DIRECTION('ref_axis',(-0.707106781186547,-0.707106781186547,-7.8504622934189E-16));
#12720=DIRECTION('center_axis',(2.22734643137795E-17,1.,1.11022302462516E-15));
#12721=DIRECTION('ref_axis',(-1.,2.22734643137795E-17,2.50823714187942E-32));
#12722=DIRECTION('center_axis',(-3.53858499469356E-34,1.11022302462516E-15,
-1.));
#12723=DIRECTION('ref_axis',(0.707106781186548,-0.707106781186547,-7.8504622934189E-16));
#12724=DIRECTION('center_axis',(-1.,-2.77555756156289E-17,-3.04610206107265E-32));
#12725=DIRECTION('ref_axis',(2.77555756156289E-17,-1.,-1.11022302462516E-15));
#12726=DIRECTION('center_axis',(2.22734643137795E-17,1.,1.11022302462516E-15));
#12727=DIRECTION('ref_axis',(3.53858499469358E-34,-1.11022302462516E-15,
1.));
#12728=DIRECTION('center_axis',(-3.53858499469356E-34,1.11022302462516E-15,
-1.));
#12729=DIRECTION('ref_axis',(0.707106781186548,-0.707106781186547,-7.8504622934189E-16));
#12730=DIRECTION('center_axis',(-1.,-2.77555756156289E-17,-3.04610206107265E-32));
#12731=DIRECTION('ref_axis',(1.96261557335472E-17,-0.707106781186549,0.707106781186546));
#12732=DIRECTION('center_axis',(2.22734643137795E-17,1.,1.11022302462516E-15));
#12733=DIRECTION('ref_axis',(3.53858499469358E-34,-1.11022302462516E-15,
1.));
#12734=DIRECTION('center_axis',(-3.53858499469356E-34,1.11022302462516E-15,
-1.));
#12735=DIRECTION('ref_axis',(1.,2.77555756156289E-17,3.04610206107265E-32));
#12736=DIRECTION('center_axis',(-1.,-2.77555756156289E-17,-3.04610206107265E-32));
#12737=DIRECTION('ref_axis',(1.96261557335472E-17,-0.707106781186549,0.707106781186546));
#12738=DIRECTION('center_axis',(2.22734643137795E-17,1.,1.11022302462516E-15));
#12739=DIRECTION('ref_axis',(0.707106781186548,-8.0079594699868E-16,0.707106781186547));
#12740=DIRECTION('center_axis',(-3.53858499469356E-34,1.11022302462516E-15,
-1.));
#12741=DIRECTION('ref_axis',(1.,2.77555756156289E-17,3.04610206107265E-32));
#12742=DIRECTION('center_axis',(1.,2.77555756156289E-17,3.04610206107265E-32));
#12743=DIRECTION('ref_axis',(1.96261557335472E-17,-0.707106781186546,-0.707106781186549));
#12744=DIRECTION('center_axis',(2.22734643137795E-17,1.,1.11022302462516E-15));
#12745=DIRECTION('ref_axis',(-3.53858499469358E-34,1.11022302462516E-15,
-1.));
#12746=DIRECTION('center_axis',(3.53858499469356E-34,-1.11022302462516E-15,
1.));
#12747=DIRECTION('ref_axis',(-1.,-2.77555756156289E-17,-3.04610206107265E-32));
#12748=DIRECTION('center_axis',(1.,2.77555756156289E-17,3.04610206107265E-32));
#12749=DIRECTION('ref_axis',(1.96261557335472E-17,-0.707106781186546,-0.707106781186549));
#12750=DIRECTION('center_axis',(2.22734643137795E-17,1.,1.11022302462516E-15));
#12751=DIRECTION('ref_axis',(-0.707106781186546,8.00795946998682E-16,-0.707106781186549));
#12752=DIRECTION('center_axis',(3.53858499469356E-34,-1.11022302462516E-15,
1.));
#12753=DIRECTION('ref_axis',(-1.,-2.77555756156289E-17,-3.04610206107265E-32));
#12754=DIRECTION('center_axis',(1.,2.77555756156289E-17,3.04610206107265E-32));
#12755=DIRECTION('ref_axis',(2.77555756156289E-17,-1.,-1.11022302462516E-15));
#12756=DIRECTION('center_axis',(2.22734643137795E-17,1.,1.11022302462516E-15));
#12757=DIRECTION('ref_axis',(-0.707106781186546,8.00795946998682E-16,-0.707106781186549));
#12758=DIRECTION('center_axis',(3.53858499469356E-34,-1.11022302462516E-15,
1.));
#12759=DIRECTION('ref_axis',(-0.707106781186547,-0.707106781186548,-7.85046229341891E-16));
#12760=DIRECTION('center_axis',(1.,2.77555756156289E-17,3.04610206107265E-32));
#12761=DIRECTION('ref_axis',(2.77555756156289E-17,-1.,-1.11022302462516E-15));
#12762=DIRECTION('center_axis',(3.53858499469356E-34,-1.11022302462516E-15,
1.));
#12763=DIRECTION('ref_axis',(0.707106781186549,-0.707106781186546,-7.85046229341888E-16));
#12764=DIRECTION('center_axis',(2.22734643137795E-17,1.,1.11022302462516E-15));
#12765=DIRECTION('ref_axis',(1.,-2.22734643137795E-17,-2.50823714187942E-32));
#12766=DIRECTION('center_axis',(-1.,-2.77555756156289E-17,-3.04610206107265E-32));
#12767=DIRECTION('ref_axis',(-3.53858499469356E-34,1.11022302462516E-15,
-1.));
#12768=DIRECTION('center_axis',(3.53858499469356E-34,-1.11022302462516E-15,
1.));
#12769=DIRECTION('ref_axis',(0.707106781186549,-0.707106781186546,-7.85046229341888E-16));
#12770=DIRECTION('center_axis',(2.22734643137795E-17,1.,1.11022302462516E-15));
#12771=DIRECTION('ref_axis',(0.707106781186548,7.692965116851E-16,-0.707106781186548));
#12772=DIRECTION('center_axis',(-1.,-2.77555756156289E-17,-3.04610206107265E-32));
#12773=DIRECTION('ref_axis',(-3.53858499469356E-34,1.11022302462516E-15,
-1.));
#12774=DIRECTION('center_axis',(3.53858499469356E-34,-1.11022302462516E-15,
1.));
#12775=DIRECTION('ref_axis',(-2.22734643137795E-17,-1.,-1.11022302462516E-15));
#12776=DIRECTION('center_axis',(2.22734643137795E-17,1.,1.11022302462516E-15));
#12777=DIRECTION('ref_axis',(0.707106781186548,7.692965116851E-16,-0.707106781186548));
#12778=DIRECTION('center_axis',(-1.,-2.77555756156289E-17,-3.04610206107265E-32));
#12779=DIRECTION('ref_axis',(1.96261557335472E-17,-0.707106781186548,-0.707106781186547));
#12780=DIRECTION('center_axis',(3.53858499469356E-34,-1.11022302462516E-15,
1.));
#12781=DIRECTION('ref_axis',(-2.22734643137795E-17,-1.,-1.11022302462516E-15));
#12782=DIRECTION('center_axis',(2.22734643137795E-17,1.,1.11022302462516E-15));
#12783=DIRECTION('ref_axis',(1.,-2.22734643137795E-17,-2.50823714187942E-32));
#12784=DIRECTION('center_axis',(-1.,-2.77555756156289E-17,-3.04610206107265E-32));
#12785=DIRECTION('ref_axis',(1.96261557335472E-17,-0.707106781186548,-0.707106781186547));
#12786=DIRECTION('center_axis',(-2.22734643137795E-17,-1.,-1.11022302462516E-15));
#12787=DIRECTION('ref_axis',(0.707106781186547,7.692965116851E-16,-0.707106781186547));
#12788=DIRECTION('center_axis',(-2.22734643137795E-17,-1.,-1.11022302462516E-15));
#12789=DIRECTION('ref_axis',(0.707106781186548,7.692965116851E-16,-0.707106781186548));
#12790=DIRECTION('',(-2.22734643137795E-17,-1.,-1.11022302462516E-15));
#12791=DIRECTION('',(2.22734643137795E-17,1.,1.11022302462516E-15));
#12792=DIRECTION('center_axis',(2.22734643137795E-17,1.,1.11022302462516E-15));
#12793=DIRECTION('ref_axis',(-3.53858499469358E-34,1.11022302462516E-15,
-1.));
#12794=DIRECTION('center_axis',(3.53858499469356E-34,-1.11022302462516E-15,
1.));
#12795=DIRECTION('ref_axis',(-0.707106781186547,-0.707106781186548,-7.85046229341891E-16));
#12796=DIRECTION('center_axis',(-2.22734643137795E-17,-1.,-1.11022302462516E-15));
#12797=DIRECTION('ref_axis',(-0.707106781186549,8.00795946998678E-16,-0.707106781186546));
#12798=DIRECTION('center_axis',(-2.22734643137795E-17,-1.,-1.11022302462516E-15));
#12799=DIRECTION('ref_axis',(-0.707106781186549,8.00795946998678E-16,-0.707106781186546));
#12800=DIRECTION('',(-2.22734643137795E-17,-1.,-1.11022302462516E-15));
#12801=DIRECTION('',(2.22734643137795E-17,1.,1.11022302462516E-15));
#12802=DIRECTION('center_axis',(1.,2.77555756156289E-17,3.04610206107265E-32));
#12803=DIRECTION('ref_axis',(1.96261557335472E-17,-0.707106781186548,-0.707106781186547));
#12804=DIRECTION('',(-1.,-2.77555756156289E-17,-3.04610206107265E-32));
#12805=DIRECTION('',(1.,2.77555756156289E-17,3.04610206107265E-32));
#12806=DIRECTION('center_axis',(-1.,-2.77555756156289E-17,-3.04610206107265E-32));
#12807=DIRECTION('ref_axis',(2.77555756156289E-17,-1.,-1.11022302462516E-15));
#12808=DIRECTION('center_axis',(2.22734643137795E-17,1.,1.11022302462516E-15));
#12809=DIRECTION('ref_axis',(0.707106781186548,-8.0079594699868E-16,0.707106781186547));
#12810=DIRECTION('center_axis',(-2.22734643137795E-17,-1.,-1.11022302462516E-15));
#12811=DIRECTION('ref_axis',(0.707106781186548,-8.0079594699868E-16,0.707106781186547));
#12812=DIRECTION('center_axis',(-2.22734643137795E-17,-1.,-1.11022302462516E-15));
#12813=DIRECTION('ref_axis',(0.707106781186548,-8.0079594699868E-16,0.707106781186547));
#12814=DIRECTION('',(-2.22734643137795E-17,-1.,-1.11022302462516E-15));
#12815=DIRECTION('',(2.22734643137795E-17,1.,1.11022302462516E-15));
#12816=DIRECTION('center_axis',(1.,2.77555756156289E-17,3.04610206107265E-32));
#12817=DIRECTION('ref_axis',(3.53858499469356E-34,-1.11022302462516E-15,
1.));
#12818=DIRECTION('center_axis',(-3.53858499469356E-34,1.11022302462516E-15,
-1.));
#12819=DIRECTION('ref_axis',(-0.707106781186547,-0.707106781186547,-7.8504622934189E-16));
#12820=DIRECTION('center_axis',(-2.22734643137795E-17,-1.,-1.11022302462516E-15));
#12821=DIRECTION('ref_axis',(-0.707106781186547,-7.69296511685101E-16,0.707106781186548));
#12822=DIRECTION('center_axis',(-2.22734643137795E-17,-1.,-1.11022302462516E-15));
#12823=DIRECTION('ref_axis',(-0.707106781186547,-7.69296511685101E-16,0.707106781186548));
#12824=DIRECTION('',(-2.22734643137795E-17,-1.,-1.11022302462516E-15));
#12825=DIRECTION('',(2.22734643137795E-17,1.,1.11022302462516E-15));
#12826=DIRECTION('center_axis',(-3.53858499469356E-34,1.11022302462516E-15,
-1.));
#12827=DIRECTION('ref_axis',(-0.707106781186547,-0.707106781186547,-7.8504622934189E-16));
#12828=DIRECTION('',(3.53858499469356E-34,-1.11022302462516E-15,1.));
#12829=DIRECTION('',(-3.53858499469356E-34,1.11022302462516E-15,-1.));
#12830=DIRECTION('center_axis',(-1.,-2.77555756156289E-17,-3.04610206107265E-32));
#12831=DIRECTION('ref_axis',(1.96261557335472E-17,-0.707106781186549,0.707106781186546));
#12832=DIRECTION('',(1.,2.77555756156289E-17,3.04610206107265E-32));
#12833=DIRECTION('',(-1.,-2.77555756156289E-17,-3.04610206107265E-32));
#12834=DIRECTION('center_axis',(3.53858499469356E-34,-1.11022302462516E-15,
1.));
#12835=DIRECTION('ref_axis',(0.707106781186549,-0.707106781186546,-7.85046229341888E-16));
#12836=DIRECTION('',(-3.53858499469356E-34,1.11022302462516E-15,-1.));
#12837=DIRECTION('',(3.53858499469356E-34,-1.11022302462516E-15,1.));
#12838=DIRECTION('center_axis',(-3.53858499469356E-34,1.11022302462516E-15,
-1.));
#12839=DIRECTION('ref_axis',(1.,2.77555756156289E-17,3.04610206107265E-32));
#12840=DIRECTION('',(-1.,-2.77555756156289E-17,-3.04610206107265E-32));
#12841=DIRECTION('',(-2.22734643137795E-17,-1.,-1.11022302462516E-15));
#12842=DIRECTION('center_axis',(3.53858499469356E-34,-1.11022302462516E-15,
1.));
#12843=DIRECTION('ref_axis',(1.,2.77555756156289E-17,3.04610206107265E-32));
#12844=DIRECTION('',(2.22734643137795E-17,1.,1.11022302462516E-15));
#12845=DIRECTION('',(-1.,-2.77555756156289E-17,-3.04610206107265E-32));
#12846=DIRECTION('',(2.22734643137795E-17,1.,1.11022302462516E-15));
#12847=DIRECTION('center_axis',(3.53858499469356E-34,-1.11022302462516E-15,
1.));
#12848=DIRECTION('ref_axis',(1.,2.77555756156289E-17,3.04610206107265E-32));
#12849=DIRECTION('',(2.22734643137795E-17,1.,1.11022302462516E-15));
#12850=DIRECTION('',(1.,2.77555756156289E-17,3.04610206107265E-32));
#12851=DIRECTION('center_axis',(2.22734643137795E-17,1.,1.11022302462516E-15));
#12852=DIRECTION('ref_axis',(1.,-2.22734643137795E-17,-2.50823714187942E-32));
#12853=DIRECTION('',(-3.53858499469356E-34,1.11022302462516E-15,-1.));
#12854=DIRECTION('',(1.,2.77555756156289E-17,3.04610206107265E-32));
#12855=DIRECTION('',(3.53858499469356E-34,-1.11022302462516E-15,1.));
#12856=DIRECTION('',(1.,2.77555756156289E-17,3.04610206107265E-32));
#12857=DIRECTION('',(-3.53858499469356E-34,1.11022302462516E-15,-1.));
#12858=DIRECTION('center_axis',(-1.,-2.77555756156289E-17,-3.04610206107265E-32));
#12859=DIRECTION('ref_axis',(-2.77555756156289E-17,1.,1.11022302462516E-15));
#12860=DIRECTION('',(-3.53858499469356E-34,1.11022302462516E-15,-1.));
#12861=DIRECTION('',(2.22734643137795E-17,1.,1.11022302462516E-15));
#12862=DIRECTION('',(3.53858499469356E-34,-1.11022302462516E-15,1.));
#12863=DIRECTION('',(2.22734643137795E-17,1.,1.11022302462516E-15));
#12864=DIRECTION('',(-3.53858499469356E-34,1.11022302462516E-15,-1.));
#12865=DIRECTION('',(2.22734643137795E-17,1.,1.11022302462516E-15));
#12866=DIRECTION('',(3.53858499469356E-34,-1.11022302462516E-15,1.));
#12867=DIRECTION('',(2.22734643137795E-17,1.,1.11022302462516E-15));
#12868=DIRECTION('center_axis',(2.22734643137795E-17,1.,1.11022302462516E-15));
#12869=DIRECTION('ref_axis',(1.,-2.22734643137795E-17,-2.50823714187942E-32));
#12870=DIRECTION('',(-1.,-2.77555756156289E-17,-3.04610206107265E-32));
#12871=DIRECTION('',(3.53858499469356E-34,-1.11022302462516E-15,1.));
#12872=DIRECTION('',(1.,2.77555756156289E-17,3.04610206107265E-32));
#12873=DIRECTION('',(3.53858499469356E-34,-1.11022302462516E-15,1.));
#12874=DIRECTION('',(-1.,-2.77555756156289E-17,-3.04610206107265E-32));
#12875=DIRECTION('center_axis',(2.22734643137795E-17,1.,1.11022302462516E-15));
#12876=DIRECTION('ref_axis',(1.,-2.22734643137795E-17,-2.50823714187942E-32));
#12877=DIRECTION('center_axis',(-2.22734643137795E-17,-1.,-1.11022302462516E-15));
#12878=DIRECTION('ref_axis',(1.,-2.22734643137795E-17,-2.50823714187942E-32));
#12879=DIRECTION('center_axis',(2.22734643137795E-17,1.,1.11022302462516E-15));
#12880=DIRECTION('ref_axis',(1.,-2.22734643137795E-17,-2.50823714187942E-32));
#12881=DIRECTION('center_axis',(-3.53858499469356E-34,1.11022302462516E-15,
-1.));
#12882=DIRECTION('ref_axis',(0.707106781186547,0.707106781186548,7.85046229341891E-16));
#12883=DIRECTION('center_axis',(3.53858499469356E-34,-1.11022302462516E-15,
1.));
#12884=DIRECTION('ref_axis',(0.707106781186547,0.707106781186548,7.85046229341891E-16));
#12885=DIRECTION('',(3.53858499469356E-34,-1.11022302462516E-15,1.));
#12886=DIRECTION('center_axis',(-3.53858499469356E-34,1.11022302462516E-15,
-1.));
#12887=DIRECTION('ref_axis',(0.707106781186547,0.707106781186548,7.85046229341891E-16));
#12888=DIRECTION('',(-3.53858499469356E-34,1.11022302462516E-15,-1.));
#12889=DIRECTION('center_axis',(2.22734643137795E-17,1.,1.11022302462516E-15));
#12890=DIRECTION('ref_axis',(1.,-2.22734643137795E-17,-2.50823714187942E-32));
#12891=DIRECTION('',(-1.,-2.77555756156289E-17,-3.04610206107265E-32));
#12892=DIRECTION('',(1.,2.77555756156289E-17,3.04610206107265E-32));
#12893=DIRECTION('center_axis',(-3.53858499469356E-34,1.11022302462516E-15,
-1.));
#12894=DIRECTION('ref_axis',(1.,2.77555756156289E-17,3.04610206107265E-32));
#12895=DIRECTION('',(2.22734643137795E-17,1.,1.11022302462516E-15));
#12896=DIRECTION('',(-1.,-2.77555756156289E-17,-3.04610206107265E-32));
#12897=DIRECTION('',(1.,2.77555756156289E-17,3.04610206107265E-32));
#12898=DIRECTION('center_axis',(-3.53858499469356E-34,1.11022302462516E-15,
-1.));
#12899=DIRECTION('ref_axis',(0.707106781186547,0.707106781186548,7.85046229341891E-16));
#12900=DIRECTION('center_axis',(3.53858499469356E-34,-1.11022302462516E-15,
1.));
#12901=DIRECTION('ref_axis',(0.707106781186547,0.707106781186548,7.85046229341891E-16));
#12902=DIRECTION('',(3.53858499469356E-34,-1.11022302462516E-15,1.));
#12903=DIRECTION('center_axis',(-3.53858499469356E-34,1.11022302462516E-15,
-1.));
#12904=DIRECTION('ref_axis',(0.707106781186547,0.707106781186548,7.85046229341891E-16));
#12905=DIRECTION('',(-3.53858499469356E-34,1.11022302462516E-15,-1.));
#12906=DIRECTION('center_axis',(2.22734643137795E-17,1.,1.11022302462516E-15));
#12907=DIRECTION('ref_axis',(1.,-2.22734643137795E-17,-2.50823714187942E-32));
#12908=DIRECTION('',(-1.,-2.77555756156289E-17,-3.04610206107265E-32));
#12909=DIRECTION('',(1.,2.77555756156289E-17,3.04610206107265E-32));
#12910=DIRECTION('center_axis',(-3.53858499469356E-34,1.11022302462516E-15,
-1.));
#12911=DIRECTION('ref_axis',(1.,2.77555756156289E-17,3.04610206107265E-32));
#12912=DIRECTION('',(2.22734643137795E-17,1.,1.11022302462516E-15));
#12913=DIRECTION('',(1.,2.77555756156289E-17,3.04610206107265E-32));
#12914=DIRECTION('center_axis',(1.,2.77555756156289E-17,3.04610206107265E-32));
#12915=DIRECTION('ref_axis',(-1.96261557335472E-17,0.707106781186547,0.707106781186549));
#12916=DIRECTION('center_axis',(-1.,-2.77555756156289E-17,-3.04610206107265E-32));
#12917=DIRECTION('ref_axis',(-1.96261557335472E-17,0.707106781186547,0.707106781186549));
#12918=DIRECTION('',(-1.,-2.77555756156289E-17,-3.04610206107265E-32));
#12919=DIRECTION('center_axis',(1.,2.77555756156289E-17,3.04610206107265E-32));
#12920=DIRECTION('ref_axis',(-1.96261557335472E-17,0.707106781186547,0.707106781186549));
#12921=DIRECTION('',(1.,2.77555756156289E-17,3.04610206107265E-32));
#12922=DIRECTION('center_axis',(-1.,-2.77555756156289E-17,-3.04610206107265E-32));
#12923=DIRECTION('ref_axis',(-2.77555756156289E-17,1.,1.11022302462516E-15));
#12924=DIRECTION('',(3.53858499469356E-34,-1.11022302462516E-15,1.));
#12925=DIRECTION('',(-3.53858499469356E-34,1.11022302462516E-15,-1.));
#12926=DIRECTION('',(2.22734643137795E-17,1.,1.11022302462516E-15));
#12927=DIRECTION('',(3.53858499469356E-34,-1.11022302462516E-15,1.));
#12928=DIRECTION('',(2.22734643137795E-17,1.,1.11022302462516E-15));
#12929=DIRECTION('center_axis',(2.22734643137795E-17,1.,1.11022302462516E-15));
#12930=DIRECTION('ref_axis',(1.,-2.22734643137795E-17,-2.50823714187942E-32));
#12931=DIRECTION('',(-3.53858499469356E-34,1.11022302462516E-15,-1.));
#12932=DIRECTION('center_axis',(-1.,-2.77555756156289E-17,-3.04610206107265E-32));
#12933=DIRECTION('ref_axis',(-1.96261557335472E-17,0.707106781186549,-0.707106781186546));
#12934=DIRECTION('center_axis',(1.,2.77555756156289E-17,3.04610206107265E-32));
#12935=DIRECTION('ref_axis',(-1.96261557335472E-17,0.707106781186549,-0.707106781186546));
#12936=DIRECTION('',(1.,2.77555756156289E-17,3.04610206107265E-32));
#12937=DIRECTION('center_axis',(-1.,-2.77555756156289E-17,-3.04610206107265E-32));
#12938=DIRECTION('ref_axis',(-1.96261557335472E-17,0.707106781186549,-0.707106781186546));
#12939=DIRECTION('',(-1.,-2.77555756156289E-17,-3.04610206107265E-32));
#12940=DIRECTION('center_axis',(1.,2.77555756156289E-17,3.04610206107265E-32));
#12941=DIRECTION('ref_axis',(-3.53858499469356E-34,1.11022302462516E-15,
-1.));
#12942=DIRECTION('',(-3.53858499469356E-34,1.11022302462516E-15,-1.));
#12943=DIRECTION('',(2.22734643137795E-17,1.,1.11022302462516E-15));
#12944=DIRECTION('',(3.53858499469356E-34,-1.11022302462516E-15,1.));
#12945=DIRECTION('',(2.22734643137795E-17,1.,1.11022302462516E-15));
#12946=DIRECTION('',(3.53858499469356E-34,-1.11022302462516E-15,1.));
#12947=DIRECTION('',(2.22734643137795E-17,1.,1.11022302462516E-15));
#12948=DIRECTION('center_axis',(2.22734643137795E-17,1.,1.11022302462516E-15));
#12949=DIRECTION('ref_axis',(1.,-2.22734643137795E-17,-2.50823714187942E-32));
#12950=DIRECTION('',(3.53858499469356E-34,-1.11022302462516E-15,1.));
#12951=DIRECTION('',(1.,2.77555756156289E-17,3.04610206107265E-32));
#12952=DIRECTION('center_axis',(3.53858499469356E-34,-1.11022302462516E-15,
1.));
#12953=DIRECTION('ref_axis',(-0.707106781186546,0.707106781186549,7.85046229341892E-16));
#12954=DIRECTION('center_axis',(-3.53858499469356E-34,1.11022302462516E-15,
-1.));
#12955=DIRECTION('ref_axis',(-0.707106781186546,0.707106781186549,7.85046229341892E-16));
#12956=DIRECTION('',(-3.53858499469356E-34,1.11022302462516E-15,-1.));
#12957=DIRECTION('center_axis',(3.53858499469356E-34,-1.11022302462516E-15,
1.));
#12958=DIRECTION('ref_axis',(-0.707106781186546,0.707106781186549,7.85046229341892E-16));
#12959=DIRECTION('',(3.53858499469356E-34,-1.11022302462516E-15,1.));
#12960=DIRECTION('center_axis',(2.22734643137795E-17,1.,1.11022302462516E-15));
#12961=DIRECTION('ref_axis',(1.,-2.22734643137795E-17,-2.50823714187942E-32));
#12962=DIRECTION('',(1.,2.77555756156289E-17,3.04610206107265E-32));
#12963=DIRECTION('',(-3.53858499469356E-34,1.11022302462516E-15,-1.));
#12964=DIRECTION('',(-1.,-2.77555756156289E-17,-3.04610206107265E-32));
#12965=DIRECTION('center_axis',(3.53858499469356E-34,-1.11022302462516E-15,
1.));
#12966=DIRECTION('ref_axis',(-2.22734643137795E-17,-1.,-1.11022302462516E-15));
#12967=DIRECTION('',(2.22734643137795E-17,1.,1.11022302462516E-15));
#12968=DIRECTION('',(-1.,-2.77555756156289E-17,-3.04610206107265E-32));
#12969=DIRECTION('',(-1.,-2.77555756156289E-17,-3.04610206107265E-32));
#12970=DIRECTION('',(2.22734643137795E-17,1.,1.11022302462516E-15));
#12971=DIRECTION('center_axis',(2.22734643137795E-17,1.,1.11022302462516E-15));
#12972=DIRECTION('ref_axis',(1.,-2.22734643137795E-17,-2.50823714187942E-32));
#12973=DIRECTION('',(-3.53858499469356E-34,1.11022302462516E-15,-1.));
#12974=DIRECTION('',(-3.53858499469356E-34,1.11022302462516E-15,-1.));
#12975=DIRECTION('',(1.,2.77555756156289E-17,3.04610206107265E-32));
#12976=DIRECTION('center_axis',(-1.,-2.77555756156289E-17,-3.04610206107265E-32));
#12977=DIRECTION('ref_axis',(-2.77555756156289E-17,1.,1.11022302462516E-15));
#12978=DIRECTION('',(2.22734643137795E-17,1.,1.11022302462516E-15));
#12979=DIRECTION('center_axis',(-3.53858499469356E-34,1.11022302462516E-15,
-1.));
#12980=DIRECTION('ref_axis',(1.,2.77555756156289E-17,3.04610206107265E-32));
#12981=DIRECTION('',(2.22734643137795E-17,1.,1.11022302462516E-15));
#12982=DIRECTION('',(1.,2.77555756156289E-17,3.04610206107265E-32));
#12983=DIRECTION('center_axis',(2.22734643137795E-17,1.,1.11022302462516E-15));
#12984=DIRECTION('ref_axis',(1.,-2.22734643137795E-17,-2.50823714187942E-32));
#12985=DIRECTION('',(3.53858499469356E-34,-1.11022302462516E-15,1.));
#12986=DIRECTION('',(-3.53858499469356E-34,1.11022302462516E-15,-1.));
#12987=DIRECTION('',(1.,2.77555756156289E-17,3.04610206107265E-32));
#12988=DIRECTION('',(3.53858499469356E-34,-1.11022302462516E-15,1.));
#12989=DIRECTION('',(1.,2.77555756156289E-17,3.04610206107265E-32));
#12990=DIRECTION('center_axis',(2.22734643137795E-17,1.,1.11022302462516E-15));
#12991=DIRECTION('ref_axis',(1.,-2.22734643137795E-17,-2.50823714187942E-32));
#12992=DIRECTION('',(-3.53858499469356E-34,1.11022302462516E-15,-1.));
#12993=DIRECTION('',(1.,2.77555756156289E-17,3.04610206107265E-32));
#12994=DIRECTION('',(-3.53858499469356E-34,1.11022302462516E-15,-1.));
#12995=DIRECTION('',(3.53858499469356E-34,-1.11022302462516E-15,1.));
#12996=DIRECTION('center_axis',(1.,2.77555756156289E-17,3.04610206107265E-32));
#12997=DIRECTION('ref_axis',(-3.53858499469356E-34,1.11022302462516E-15,
-1.));
#12998=DIRECTION('',(2.22734643137795E-17,1.,1.11022302462516E-15));
#12999=DIRECTION('',(-3.53858499469356E-34,1.11022302462516E-15,-1.));
#13000=DIRECTION('center_axis',(3.53858499469356E-34,-1.11022302462516E-15,
1.));
#13001=DIRECTION('ref_axis',(-2.22734643137795E-17,-1.,-1.11022302462516E-15));
#13002=DIRECTION('',(1.,2.77555756156289E-17,3.04610206107265E-32));
#13003=DIRECTION('center_axis',(2.22734643137795E-17,1.,1.11022302462516E-15));
#13004=DIRECTION('ref_axis',(1.,-2.22734643137795E-17,-2.50823714187942E-32));
#13005=DIRECTION('',(3.53858499469356E-34,-1.11022302462516E-15,1.));
#13006=DIRECTION('center_axis',(2.22734643137795E-17,1.,1.11022302462516E-15));
#13007=DIRECTION('ref_axis',(1.,-2.22734643137795E-17,-2.50823714187942E-32));
#13008=DIRECTION('',(3.53858499469356E-34,-1.11022302462516E-15,1.));
#13009=DIRECTION('',(-1.,-2.77555756156289E-17,-3.04610206107265E-32));
#13010=DIRECTION('center_axis',(-3.53858499469356E-34,1.11022302462516E-15,
-1.));
#13011=DIRECTION('ref_axis',(1.,2.77555756156289E-17,3.04610206107265E-32));
#13012=DIRECTION('',(1.,2.77555756156289E-17,3.04610206107265E-32));
#13013=DIRECTION('',(2.22734643137795E-17,1.,1.11022302462516E-15));
#13014=DIRECTION('center_axis',(2.22734643137795E-17,1.,1.11022302462516E-15));
#13015=DIRECTION('ref_axis',(1.,-2.22734643137795E-17,-2.50823714187942E-32));
#13016=DIRECTION('',(1.,2.77555756156289E-17,3.04610206107265E-32));
#13017=DIRECTION('',(-3.53858499469356E-34,1.11022302462516E-15,-1.));
#13018=DIRECTION('center_axis',(2.22734643137795E-17,1.,1.11022302462516E-15));
#13019=DIRECTION('ref_axis',(1.,-2.22734643137795E-17,-2.50823714187942E-32));
#13020=DIRECTION('',(3.53858499469356E-34,-1.11022302462516E-15,1.));
#13021=DIRECTION('',(3.53858499469356E-34,-1.11022302462516E-15,1.));
#13022=DIRECTION('',(-1.,-2.77555756156289E-17,-3.04610206107265E-32));
#13023=DIRECTION('center_axis',(1.,2.77555756156289E-17,3.04610206107265E-32));
#13024=DIRECTION('ref_axis',(-3.53858499469356E-34,1.11022302462516E-15,
-1.));
#13025=DIRECTION('',(2.22734643137795E-17,1.,1.11022302462516E-15));
#13026=DIRECTION('center_axis',(3.53858499469356E-34,-1.11022302462516E-15,
1.));
#13027=DIRECTION('ref_axis',(-2.22734643137795E-17,-1.,-1.11022302462516E-15));
#13028=DIRECTION('center_axis',(3.53858499469356E-34,-1.11022302462516E-15,
1.));
#13029=DIRECTION('ref_axis',(-2.22734643137795E-17,-1.,-1.11022302462516E-15));
#13030=DIRECTION('',(1.,2.77555756156289E-17,3.04610206107265E-32));
#13031=DIRECTION('',(2.22734643137795E-17,1.,1.11022302462516E-15));
#13032=DIRECTION('center_axis',(2.22734643137795E-17,1.,1.11022302462516E-15));
#13033=DIRECTION('ref_axis',(1.,-2.22734643137795E-17,-2.50823714187942E-32));
#13034=DIRECTION('',(1.,2.77555756156289E-17,3.04610206107265E-32));
#13035=DIRECTION('',(-3.53858499469356E-34,1.11022302462516E-15,-1.));
#13036=DIRECTION('center_axis',(2.22734643137795E-17,1.,1.11022302462516E-15));
#13037=DIRECTION('ref_axis',(1.,0.,0.));
#13038=DIRECTION('center_axis',(0.,1.11022302462516E-15,-1.));
#13039=DIRECTION('ref_axis',(-1.,0.,0.));
#13040=DIRECTION('center_axis',(-2.22734643137795E-17,-1.,-1.11022302462516E-15));
#13041=DIRECTION('ref_axis',(1.,-2.22734643137795E-17,-2.50823714187942E-32));
#13042=DIRECTION('center_axis',(-2.22734643137795E-17,-1.,-1.11022302462516E-15));
#13043=DIRECTION('ref_axis',(1.,-2.22734643137795E-17,-2.50823714187942E-32));
#13044=DIRECTION('center_axis',(-2.22734643137795E-17,-1.,-1.11022302462516E-15));
#13045=DIRECTION('ref_axis',(1.,-2.22734643137795E-17,-2.50823714187942E-32));
#13046=DIRECTION('',(-2.22734643137795E-17,-1.,-1.11022302462516E-15));
#13047=DIRECTION('center_axis',(2.22734643137795E-17,1.,1.11022302462516E-15));
#13048=DIRECTION('ref_axis',(1.,-2.22734643137795E-17,-2.50823714187942E-32));
#13049=DIRECTION('center_axis',(-2.22734643137795E-17,-1.,-1.11022302462516E-15));
#13050=DIRECTION('ref_axis',(3.53858499469358E-34,-1.11022302462516E-15,
1.));
#13051=DIRECTION('center_axis',(2.22734643137795E-17,1.,1.11022302462516E-15));
#13052=DIRECTION('ref_axis',(1.,-2.22734643137795E-17,-2.50823714187942E-32));
#13053=DIRECTION('center_axis',(-2.22734643137795E-17,-1.,-1.11022302462516E-15));
#13054=DIRECTION('ref_axis',(1.,-2.22734643137795E-17,-2.50823714187942E-32));
#13055=DIRECTION('',(-3.53858499469356E-34,1.11022302462516E-15,-1.));
#13056=DIRECTION('',(-1.,-2.77555756156289E-17,-3.04610206107265E-32));
#13057=DIRECTION('',(3.53858499469356E-34,-1.11022302462516E-15,1.));
#13058=DIRECTION('',(-1.,-2.77555756156289E-17,-3.04610206107265E-32));
#13059=DIRECTION('',(-3.53858499469356E-34,1.11022302462516E-15,-1.));
#13060=DIRECTION('center_axis',(-2.22734643137795E-17,-1.,-1.11022302462516E-15));
#13061=DIRECTION('ref_axis',(1.,-2.22734643137795E-17,-2.50823714187942E-32));
#13062=DIRECTION('',(-2.22734643137795E-17,-1.,-1.11022302462516E-15));
#13063=DIRECTION('center_axis',(1.,2.77555756156289E-17,3.04610206107265E-32));
#13064=DIRECTION('ref_axis',(-3.53858499469356E-34,1.11022302462516E-15,
-1.));
#13065=DIRECTION('',(-2.22734643137795E-17,-1.,-1.11022302462516E-15));
#13066=DIRECTION('',(-2.22734643137795E-17,-1.,-1.11022302462516E-15));
#13067=DIRECTION('center_axis',(1.,2.77555756156289E-17,3.04610206107265E-32));
#13068=DIRECTION('ref_axis',(-3.53858499469356E-34,1.11022302462516E-15,
-1.));
#13069=DIRECTION('center_axis',(3.53858499469356E-34,-1.11022302462516E-15,
1.));
#13070=DIRECTION('ref_axis',(-2.22734643137795E-17,-1.,-1.11022302462516E-15));
#13071=DIRECTION('',(-2.22734643137795E-17,-1.,-1.11022302462516E-15));
#13072=DIRECTION('center_axis',(3.53858499469356E-34,-1.11022302462516E-15,
1.));
#13073=DIRECTION('ref_axis',(1.,2.77555756156289E-17,3.04610206107265E-32));
#13074=DIRECTION('',(-2.22734643137795E-17,-1.,-1.11022302462516E-15));
#13075=DIRECTION('',(2.22734643137795E-17,1.,1.11022302462516E-15));
#13076=DIRECTION('',(2.22734643137795E-17,1.,1.11022302462516E-15));
#13077=DIRECTION('center_axis',(3.53858499469356E-34,-1.11022302462516E-15,
1.));
#13078=DIRECTION('ref_axis',(1.,2.77555756156289E-17,3.04610206107265E-32));
#13079=DIRECTION('center_axis',(1.,2.77555756156289E-17,3.04610206107265E-32));
#13080=DIRECTION('ref_axis',(-3.53858499469356E-34,1.11022302462516E-15,
-1.));
#13081=DIRECTION('',(-3.53858499469356E-34,1.11022302462516E-15,-1.));
#13082=DIRECTION('center_axis',(-3.53858499469356E-34,1.11022302462516E-15,
-1.));
#13083=DIRECTION('ref_axis',(1.,2.77555756156289E-17,3.04610206107265E-32));
#13084=DIRECTION('center_axis',(1.,2.77555756156289E-17,3.04610206107265E-32));
#13085=DIRECTION('ref_axis',(-3.53858499469356E-34,1.11022302462516E-15,
-1.));
#13086=DIRECTION('',(-3.53858499469356E-34,1.11022302462516E-15,-1.));
#13087=DIRECTION('center_axis',(-1.,-2.77555756156289E-17,-3.04610206107265E-32));
#13088=DIRECTION('ref_axis',(-2.77555756156289E-17,1.,1.11022302462516E-15));
#13089=DIRECTION('',(-3.53858499469356E-34,1.11022302462516E-15,-1.));
#13090=DIRECTION('center_axis',(-3.53858499469356E-34,1.11022302462516E-15,
-1.));
#13091=DIRECTION('ref_axis',(-1.2933087539066E-15,-1.,-1.11022302462516E-15));
#13092=DIRECTION('center_axis',(-1.,-2.77555756156289E-17,-3.04610206107265E-32));
#13093=DIRECTION('ref_axis',(-2.77555756156289E-17,1.,1.11022302462516E-15));
#13094=DIRECTION('',(2.22734643137795E-17,1.,1.11022302462516E-15));
#13095=DIRECTION('center_axis',(3.53858499469356E-34,-1.11022302462516E-15,
1.));
#13096=DIRECTION('ref_axis',(-1.98232732358613E-15,-1.,-1.11022302462516E-15));
#13097=DIRECTION('center_axis',(3.53858499469356E-34,-1.11022302462516E-15,
1.));
#13098=DIRECTION('ref_axis',(1.,2.77555756156289E-17,3.04610206107265E-32));
#13099=DIRECTION('center_axis',(-3.53858499469356E-34,1.11022302462516E-15,
-1.));
#13100=DIRECTION('ref_axis',(1.,2.77555756156289E-17,3.04610206107265E-32));
#13101=DIRECTION('',(3.53858499469356E-34,-1.11022302462516E-15,1.));
#13102=DIRECTION('center_axis',(-1.,-2.77555756156289E-17,-3.04610206107265E-32));
#13103=DIRECTION('ref_axis',(-2.77555756156289E-17,1.,1.11022302462516E-15));
#13104=DIRECTION('',(2.22734643137795E-17,1.,1.11022302462516E-15));
#13105=DIRECTION('',(-2.22734643137795E-17,-1.,-1.11022302462516E-15));
#13106=DIRECTION('center_axis',(1.,2.77555756156289E-17,3.04610206107265E-32));
#13107=DIRECTION('ref_axis',(-3.53858499469356E-34,1.11022302462516E-15,
-1.));
#13108=DIRECTION('',(2.22734643137795E-17,1.,1.11022302462516E-15));
#13109=DIRECTION('',(2.22734643137795E-17,1.,1.11022302462516E-15));
#13110=DIRECTION('',(3.53858499469356E-34,-1.11022302462516E-15,1.));
#13111=DIRECTION('center_axis',(3.53858499469356E-34,-1.11022302462516E-15,
1.));
#13112=DIRECTION('ref_axis',(1.,2.77555756156289E-17,3.04610206107265E-32));
#13113=DIRECTION('center_axis',(3.53858499469356E-34,-1.11022302462516E-15,
1.));
#13114=DIRECTION('ref_axis',(1.,2.77555756156289E-17,3.04610206107265E-32));
#13115=DIRECTION('center_axis',(-3.53858499469356E-34,1.11022302462516E-15,
-1.));
#13116=DIRECTION('ref_axis',(1.,2.77555756156289E-17,3.04610206107265E-32));
#13117=DIRECTION('',(3.53858499469356E-34,-1.11022302462516E-15,1.));
#13118=DIRECTION('center_axis',(-1.,-2.77555756156289E-17,-3.04610206107265E-32));
#13119=DIRECTION('ref_axis',(-2.77555756156289E-17,1.,1.11022302462516E-15));
#13120=DIRECTION('',(2.22734643137795E-17,1.,1.11022302462516E-15));
#13121=DIRECTION('',(2.22734643137795E-17,1.,1.11022302462516E-15));
#13122=DIRECTION('center_axis',(3.53858499469356E-34,-1.11022302462516E-15,
1.));
#13123=DIRECTION('ref_axis',(-2.22734643137795E-17,-1.,-1.11022302462516E-15));
#13124=DIRECTION('center_axis',(3.53858499469356E-34,-1.11022302462516E-15,
1.));
#13125=DIRECTION('ref_axis',(-2.22734643137795E-17,-1.,-1.11022302462516E-15));
#44427=CARTESIAN_POINT('',(0.,0.,0.));
#44428=CARTESIAN_POINT('Ctrl Pts',(-0.0157884048591435,-0.0420671254389844,
-0.00338750223744593));
#44429=CARTESIAN_POINT('Ctrl Pts',(-0.0157173431715818,-0.0421026592929782,
-0.0033519683834522));
#44430=CARTESIAN_POINT('Ctrl Pts',(-0.0155636558736841,-0.0421616223021478,
-0.0032930053742826));
#44431=CARTESIAN_POINT('Ctrl Pts',(-0.015159650326158,-0.0422415979526153,
-0.00321302972381513));
#44432=CARTESIAN_POINT('Ctrl Pts',(-0.0148456426300394,-0.0422591074225579,
-0.00319552025387248));
#44433=CARTESIAN_POINT('Ctrl Pts',(-0.0147000397563992,-0.0422591044750182,
-0.00319552320141217));
#44434=CARTESIAN_POINT('Ctrl Pts',(-0.0157528787075658,-0.0421381807912534,
-0.00342302785458162));
#44435=CARTESIAN_POINT('Ctrl Pts',(-0.0156824358684872,-0.0421664366105109,
-0.00338793404912082));
#44436=CARTESIAN_POINT('Ctrl Pts',(-0.0155288204070857,-0.0422151679902414,
-0.00332877315343381));
#44437=CARTESIAN_POINT('Ctrl Pts',(-0.0151292237928858,-0.0422873985837832,
-0.00325294897397118));
#44438=CARTESIAN_POINT('Ctrl Pts',(-0.0148375584890053,-0.042302815988272,
-0.00323922980950275));
#44439=CARTESIAN_POINT('Ctrl Pts',(-0.0147000438396441,-0.0423053858040627,
-0.00324180453020668));
#44440=CARTESIAN_POINT('Ctrl Pts',(-0.0156744511200191,-0.0422592722231825,
-0.00350145526245708));
#44441=CARTESIAN_POINT('Ctrl Pts',(-0.0156040258414969,-0.0422778860192918,
-0.00346670011416197));
#44442=CARTESIAN_POINT('Ctrl Pts',(-0.0154465327860142,-0.0423135447464296,
-0.00340860687607781));
#44443=CARTESIAN_POINT('Ctrl Pts',(-0.015057946353037,-0.0423722576286869,
-0.00334646106679692));
#44444=CARTESIAN_POINT('Ctrl Pts',(-0.0148199479540628,-0.0423811726973118,
-0.00333924835453889));
#44445=CARTESIAN_POINT('Ctrl Pts',(-0.0147000527348183,-0.0423857572179057,
-0.00334654796809966));
#44446=CARTESIAN_POINT('Ctrl Pts',(-0.0154683605023745,-0.0424274066208669,
-0.00370754740791061));
#44447=CARTESIAN_POINT('Ctrl Pts',(-0.0153984617189363,-0.0424344514374246,
-0.00366923932138871));
#44448=CARTESIAN_POINT('Ctrl Pts',(-0.0152393099806225,-0.0424501760183733,
-0.0036057457320669));
#44449=CARTESIAN_POINT('Ctrl Pts',(-0.0149608392286012,-0.0424602418154941,
-0.00353217877322852));
#44450=CARTESIAN_POINT('Ctrl Pts',(-0.0147915700499568,-0.0424596290594207,
-0.00352111890571466));
#44451=CARTESIAN_POINT('Ctrl Pts',(-0.0147000670678934,-0.0424615469535684,
-0.00352952438408725));
#44452=CARTESIAN_POINT('Ctrl Pts',(-0.0153031604679818,-0.0424787830360679,
-0.00387274336261303));
#44453=CARTESIAN_POINT('Ctrl Pts',(-0.0152490565373728,-0.0424787818503424,
-0.00382672158200888));
#44454=CARTESIAN_POINT('Ctrl Pts',(-0.0151294062024839,-0.0424787792037381,
-0.00374633773382312));
#44455=CARTESIAN_POINT('Ctrl Pts',(-0.0149205641771022,-0.0424787775093944,
-0.00366927823060112));
#44456=CARTESIAN_POINT('Ctrl Pts',(-0.0147740219052253,-0.0424787776124787,
-0.00365678806556642));
#44457=CARTESIAN_POINT('Ctrl Pts',(-0.0147000759302474,-0.0424787772896768,
-0.00366042730492668));
#44458=CARTESIAN_POINT('Ctrl Pts',(-0.0152303498648171,-0.0424787743876894,
-0.00394555014548032));
#44459=CARTESIAN_POINT('Ctrl Pts',(-0.0151840750377049,-0.0424787743879888,
-0.0038992671324187));
#44460=CARTESIAN_POINT('Ctrl Pts',(-0.0150793499745268,-0.042478774388657,
-0.0038188996061916));
#44461=CARTESIAN_POINT('Ctrl Pts',(-0.0148964045588548,-0.0424787743890847,
-0.0037431163626244));
#44462=CARTESIAN_POINT('Ctrl Pts',(-0.014765526907758,-0.0424787743890587,
-0.00372588526759391));
#44463=CARTESIAN_POINT('Ctrl Pts',(-0.0147000802206811,-0.0424787743891402,
-0.00372588633138974));
#44464=CARTESIAN_POINT('',(-0.0157883689862958,-0.0420671433761681,-0.00338748430026228));
#44465=CARTESIAN_POINT('',(-0.0147001132585517,-0.0422591044757622,-0.0031955232006682));
#44466=CARTESIAN_POINT('Ctrl Pts',(-0.0157883689863059,-0.0420671433761781,
-0.00338748430025228));
#44467=CARTESIAN_POINT('Ctrl Pts',(-0.0157173173078478,-0.0421026692154071,
-0.00335195846102329));
#44468=CARTESIAN_POINT('Ctrl Pts',(-0.0155636332119379,-0.0421616267882068,
-0.00329300088822358));
#44469=CARTESIAN_POINT('Ctrl Pts',(-0.0151596729879242,-0.0422415934665763,
-0.00321303420985414));
#44470=CARTESIAN_POINT('Ctrl Pts',(-0.0148456954718,-0.0422591044757722,
-0.0031955232006582));
#44471=CARTESIAN_POINT('Ctrl Pts',(-0.0147001132585417,-0.0422591044757722,
-0.0031955232006582));
#44472=CARTESIAN_POINT('',(-0.0152303632585517,-0.0424787743898723,-0.00394549002800645));
#44473=CARTESIAN_POINT('Ctrl Pts',(-0.0157883689863059,-0.0420671433761781,
-0.00338748430025228));
#44474=CARTESIAN_POINT('Ctrl Pts',(-0.0157528431470768,-0.0421381950546361,
-0.00342301013948126));
#44475=CARTESIAN_POINT('Ctrl Pts',(-0.0156744155682287,-0.0422592816194792,
-0.00350143771832943));
#44476=CARTESIAN_POINT('Ctrl Pts',(-0.0154683367770566,-0.0424274007458997,
-0.00370751650950155));
#44477=CARTESIAN_POINT('Ctrl Pts',(-0.0153031609543063,-0.0424787743898823,
-0.00387269233225182));
#44478=CARTESIAN_POINT('Ctrl Pts',(-0.0152303632585616,-0.0424787743898823,
-0.00394549002799644));
#44479=CARTESIAN_POINT('',(-0.0147001132585517,-0.0424787743898723,-0.00372585328655811));
#44480=CARTESIAN_POINT('Origin',(-0.0147001132585417,-0.0424787743898823,
-0.00447574002801644));
#44481=CARTESIAN_POINT('Origin',(-0.0147001132585417,-0.0417287743898823,
-0.00372585328654811));
#44482=CARTESIAN_POINT('Ctrl Pts',(-0.0157883510491122,-0.0420671254389845,
-0.0033874484274146));
#44483=CARTESIAN_POINT('Ctrl Pts',(-0.0157528254319766,-0.0421381807912534,
-0.00342297457899241));
#44484=CARTESIAN_POINT('Ctrl Pts',(-0.0156743980241011,-0.0422592722231825,
-0.00350140216653908));
#44485=CARTESIAN_POINT('Ctrl Pts',(-0.0154683058786476,-0.0424274066208669,
-0.00370749278418372));
#44486=CARTESIAN_POINT('Ctrl Pts',(-0.0153031099239451,-0.042478783036068,
-0.00387269281857635));
#44487=CARTESIAN_POINT('Ctrl Pts',(-0.0152303031410779,-0.0424787743876895,
-0.00394550342174105));
#44488=CARTESIAN_POINT('Ctrl Pts',(-0.0158238849031059,-0.0421026592929782,
-0.00345851011497633));
#44489=CARTESIAN_POINT('Ctrl Pts',(-0.0157879192374373,-0.0421664366105109,
-0.00349341741807102));
#44490=CARTESIAN_POINT('Ctrl Pts',(-0.0157091531723962,-0.0422778860192918,
-0.00357182744506125));
#44491=CARTESIAN_POINT('Ctrl Pts',(-0.0155066139651694,-0.0424344514374246,
-0.00377739156762176));
#44492=CARTESIAN_POINT('Ctrl Pts',(-0.0153491317045492,-0.0424787818503424,
-0.00392679674918539));
#44493=CARTESIAN_POINT('Ctrl Pts',(-0.0152765861541394,-0.0424787743879888,
-0.00399177824885321));
#44494=CARTESIAN_POINT('Ctrl Pts',(-0.0158828479122755,-0.0421616223021478,
-0.00361219741287408));
#44495=CARTESIAN_POINT('Ctrl Pts',(-0.0158470801331243,-0.0422151679902414,
-0.00364703287947237));
#44496=CARTESIAN_POINT('Ctrl Pts',(-0.0157672464104804,-0.0423135447464296,
-0.00372932050054389));
#44497=CARTESIAN_POINT('Ctrl Pts',(-0.0155701075544912,-0.0424501760183733,
-0.0039365433059356));
#44498=CARTESIAN_POINT('Ctrl Pts',(-0.015429515552735,-0.0424787792037381,
-0.00404644708407416));
#44499=CARTESIAN_POINT('Ctrl Pts',(-0.0153569536803665,-0.042478774388657,
-0.00409650331203122));
#44500=CARTESIAN_POINT('Ctrl Pts',(-0.0159628235627429,-0.0422415979526153,
-0.00401620296040003));
#44501=CARTESIAN_POINT('Ctrl Pts',(-0.015922904312587,-0.0422873985837832,
-0.00404662949367233));
#44502=CARTESIAN_POINT('Ctrl Pts',(-0.0158293922197611,-0.0423722576286869,
-0.00411790693352109));
#44503=CARTESIAN_POINT('Ctrl Pts',(-0.0156436745133296,-0.0424602418154941,
-0.00421501405795683));
#44504=CARTESIAN_POINT('Ctrl Pts',(-0.0155065750559569,-0.0424787775093944,
-0.00425528910945595));
#44505=CARTESIAN_POINT('Ctrl Pts',(-0.0154327369239338,-0.0424787743890847,
-0.00427944872770332));
#44506=CARTESIAN_POINT('Ctrl Pts',(-0.0159803330326856,-0.0422591074225579,
-0.00433021065651868));
#44507=CARTESIAN_POINT('Ctrl Pts',(-0.0159366234770553,-0.042302815988272,
-0.00433829479755283));
#44508=CARTESIAN_POINT('Ctrl Pts',(-0.0158366049320192,-0.0423811726973118,
-0.00435590533249528));
#44509=CARTESIAN_POINT('Ctrl Pts',(-0.0156547343808434,-0.0424596290594207,
-0.0043842832366013));
#44510=CARTESIAN_POINT('Ctrl Pts',(-0.0155190652209917,-0.0424787776124787,
-0.00440183138133276));
#44511=CARTESIAN_POINT('Ctrl Pts',(-0.0154499680189642,-0.0424787743890587,
-0.00441032637880006));
#44512=CARTESIAN_POINT('Ctrl Pts',(-0.0159803300851459,-0.0422591044750182,
-0.00447581353015889));
#44513=CARTESIAN_POINT('Ctrl Pts',(-0.0159340487563514,-0.0423053858040627,
-0.004475809446914));
#44514=CARTESIAN_POINT('Ctrl Pts',(-0.0158293053184584,-0.0423857572179057,
-0.00447580055173977));
#44515=CARTESIAN_POINT('Ctrl Pts',(-0.0156463289024708,-0.0424615469535684,
-0.0044757862186647));
#44516=CARTESIAN_POINT('Ctrl Pts',(-0.0155154259816315,-0.0424787772896768,
-0.0044757773563107));
#44517=CARTESIAN_POINT('Ctrl Pts',(-0.0154499669551684,-0.0424787743891402,
-0.00447577306587701));
#44518=CARTESIAN_POINT('',(-0.0159803300858899,-0.0422591044757622,-0.00447574002800645));
#44519=CARTESIAN_POINT('Ctrl Pts',(-0.0157883689863059,-0.0420671433761781,
-0.00338748430025228));
#44520=CARTESIAN_POINT('Ctrl Pts',(-0.0158238948255348,-0.0421026692154071,
-0.00345853597871023));
#44521=CARTESIAN_POINT('Ctrl Pts',(-0.0158828523983345,-0.0421616267882069,
-0.00361222007462022));
#44522=CARTESIAN_POINT('Ctrl Pts',(-0.0159628190767039,-0.0422415934665763,
-0.00401618029863389));
#44523=CARTESIAN_POINT('Ctrl Pts',(-0.0159803300858999,-0.0422591044757722,
-0.00433015781475808));
#44524=CARTESIAN_POINT('Ctrl Pts',(-0.0159803300858999,-0.0422591044757722,
-0.00447574002801644));
#44525=CARTESIAN_POINT('',(-0.01545,-0.0424787743898723,-0.00447574002800645));
#44526=CARTESIAN_POINT('Origin',(-0.01545000000001,-0.0417287743898823,
-0.00447574002801644));
#44527=CARTESIAN_POINT('Origin',(-0.0147001132585417,-0.0424787743898823,
-0.00447574002801644));
#44528=CARTESIAN_POINT('Ctrl Pts',(-0.0157883510491121,-0.0420671254389844,
-0.00338744842741457));
#44529=CARTESIAN_POINT('Ctrl Pts',(-0.0158238849031059,-0.0421026592929782,
-0.00345851011497631));
#44530=CARTESIAN_POINT('Ctrl Pts',(-0.0158828479122755,-0.0421616223021478,
-0.00361219741287406));
#44531=CARTESIAN_POINT('Ctrl Pts',(-0.0159628235627429,-0.0422415979526153,
-0.00401620296040005));
#44532=CARTESIAN_POINT('Ctrl Pts',(-0.0159803330326856,-0.0422591074225579,
-0.00433021065651872));
#44533=CARTESIAN_POINT('Ctrl Pts',(-0.0159803300851459,-0.0422591044750182,
-0.00447581353015895));
#44534=CARTESIAN_POINT('Ctrl Pts',(-0.0158594064013811,-0.0420315998218488,
-0.00342297457899238));
#44535=CARTESIAN_POINT('Ctrl Pts',(-0.0158876622206386,-0.0420666936273096,
-0.003493417418071));
#44536=CARTESIAN_POINT('Ctrl Pts',(-0.0159363936003691,-0.0421258545229966,
-0.00364703287947235));
#44537=CARTESIAN_POINT('Ctrl Pts',(-0.0160086241939108,-0.0422016787024593,
-0.00404662949367235));
#44538=CARTESIAN_POINT('Ctrl Pts',(-0.0160240415983997,-0.0422153978669277,
-0.00433829479755287));
#44539=CARTESIAN_POINT('Ctrl Pts',(-0.0160266114141903,-0.0422128231462237,
-0.00447580944691406));
#44540=CARTESIAN_POINT('Ctrl Pts',(-0.0159804978333101,-0.0419531724139733,
-0.00350140216653905));
#44541=CARTESIAN_POINT('Ctrl Pts',(-0.0159991116294195,-0.0419879275622684,
-0.00357182744506123));
#44542=CARTESIAN_POINT('Ctrl Pts',(-0.0160347703565572,-0.0420460208003526,
-0.00372932050054387));
#44543=CARTESIAN_POINT('Ctrl Pts',(-0.0160934832388146,-0.0421081666096335,
-0.00411790693352111));
#44544=CARTESIAN_POINT('Ctrl Pts',(-0.0161023983074396,-0.0421153793218916,
-0.00435590533249531));
#44545=CARTESIAN_POINT('Ctrl Pts',(-0.0161069828280333,-0.0421080797083308,
-0.00447580055173983));
#44546=CARTESIAN_POINT('Ctrl Pts',(-0.0161486322309946,-0.0417470802685198,
-0.00370749278418369));
#44547=CARTESIAN_POINT('Ctrl Pts',(-0.0161556770475524,-0.0417853883550417,
-0.00377739156762175));
#44548=CARTESIAN_POINT('Ctrl Pts',(-0.0161714016285009,-0.0418488819443635,
-0.00393654330593559));
#44549=CARTESIAN_POINT('Ctrl Pts',(-0.0161814674256218,-0.0419224489032019,
-0.00421501405795684));
#44550=CARTESIAN_POINT('Ctrl Pts',(-0.0161808546695484,-0.0419335087707158,
-0.00438428323660133));
#44551=CARTESIAN_POINT('Ctrl Pts',(-0.0161827725636961,-0.0419251032923432,
-0.00447578621866474));
#44552=CARTESIAN_POINT('Ctrl Pts',(-0.0162000086461957,-0.0415818843138174,
-0.00387269281857635));
#44553=CARTESIAN_POINT('Ctrl Pts',(-0.0162000074604701,-0.0416279060944215,
-0.00392679674918539));
#44554=CARTESIAN_POINT('Ctrl Pts',(-0.0162000048138658,-0.0417082899426073,
-0.00404644708407417));
#44555=CARTESIAN_POINT('Ctrl Pts',(-0.0162000031195221,-0.0417853494458292,
-0.00425528910945597));
#44556=CARTESIAN_POINT('Ctrl Pts',(-0.0162000032226064,-0.041797839610864,
-0.00440183138133279));
#44557=CARTESIAN_POINT('Ctrl Pts',(-0.0162000028998045,-0.0417942003715037,
-0.00447577735631073));
#44558=CARTESIAN_POINT('Ctrl Pts',(-0.0161999999978171,-0.0415090775309501,
-0.00394550342174106));
#44559=CARTESIAN_POINT('Ctrl Pts',(-0.0161999999981165,-0.0415553605440118,
-0.00399177824885322));
#44560=CARTESIAN_POINT('Ctrl Pts',(-0.0161999999987847,-0.0416357280702388,
-0.00409650331203123));
#44561=CARTESIAN_POINT('Ctrl Pts',(-0.0161999999992124,-0.0417115113138059,
-0.00427944872770334));
#44562=CARTESIAN_POINT('Ctrl Pts',(-0.0161999999991864,-0.0417287424088365,
-0.00441032637880008));
#44563=CARTESIAN_POINT('Ctrl Pts',(-0.0161999999992679,-0.0417287413450407,
-0.00447577306587704));
#44564=CARTESIAN_POINT('',(-0.0162,-0.041509137648424,-0.00394549002800645));
#44565=CARTESIAN_POINT('Ctrl Pts',(-0.0157883689863059,-0.0420671433761781,
-0.00338748430025228));
#44566=CARTESIAN_POINT('Ctrl Pts',(-0.0158594206647638,-0.0420316175369492,
-0.00342301013948126));
#44567=CARTESIAN_POINT('Ctrl Pts',(-0.0159805072296069,-0.041953189958101,
-0.00350143771832943));
#44568=CARTESIAN_POINT('Ctrl Pts',(-0.0161486263560273,-0.0417471111669288,
-0.00370751650950155));
#44569=CARTESIAN_POINT('Ctrl Pts',(-0.01620000000001,-0.0415819353441786,
-0.00387269233225182));
#44570=CARTESIAN_POINT('Ctrl Pts',(-0.01620000000001,-0.041509137648434,
-0.00394549002799644));
#44571=CARTESIAN_POINT('',(-0.0162,-0.0417287743898723,-0.00447574002800645));
#44572=CARTESIAN_POINT('Origin',(-0.01620000000001,-0.040978887648414,-0.00447574002801644));
#44573=CARTESIAN_POINT('Origin',(-0.01545000000001,-0.0417287743898823,
-0.00447574002801644));
#44574=CARTESIAN_POINT('Ctrl Pts',(-0.0157883510491121,-0.0420671792490158,
-0.00338750223744593));
#44575=CARTESIAN_POINT('Ctrl Pts',(-0.0158594064013811,-0.0420316530974381,
-0.00342302785458162));
#44576=CARTESIAN_POINT('Ctrl Pts',(-0.0159804978333101,-0.0419532255098914,
-0.00350145526245708));
#44577=CARTESIAN_POINT('Ctrl Pts',(-0.0161486322309946,-0.0417471348922468,
-0.00370754740791061));
#44578=CARTESIAN_POINT('Ctrl Pts',(-0.0162000086461957,-0.0415819348578541,
-0.00387274336261302));
#44579=CARTESIAN_POINT('Ctrl Pts',(-0.0161999999978171,-0.0415091242546894,
-0.00394555014548031));
#44580=CARTESIAN_POINT('Ctrl Pts',(-0.0158238849031059,-0.0419961175614541,
-0.0033519683834522));
#44581=CARTESIAN_POINT('Ctrl Pts',(-0.0158876622206386,-0.0419612102583594,
-0.00338793404912082));
#44582=CARTESIAN_POINT('Ctrl Pts',(-0.0159991116294195,-0.0418828002313692,
-0.00346670011416197));
#44583=CARTESIAN_POINT('Ctrl Pts',(-0.0161556770475524,-0.0416772361088086,
-0.0036692393213887));
#44584=CARTESIAN_POINT('Ctrl Pts',(-0.0162000074604701,-0.041527830927245,
-0.00382672158200888));
#44585=CARTESIAN_POINT('Ctrl Pts',(-0.0161999999981165,-0.0414628494275772,
-0.0038992671324187));
#44586=CARTESIAN_POINT('Ctrl Pts',(-0.0158828479122755,-0.0418424302635564,
-0.0032930053742826));
#44587=CARTESIAN_POINT('Ctrl Pts',(-0.0159363936003691,-0.041807594796958,
-0.00332877315343381));
#44588=CARTESIAN_POINT('Ctrl Pts',(-0.0160347703565572,-0.0417253071758865,
-0.00340860687607781));
#44589=CARTESIAN_POINT('Ctrl Pts',(-0.0161714016285009,-0.0415180843704948,
-0.0036057457320669));
#44590=CARTESIAN_POINT('Ctrl Pts',(-0.0162000048138658,-0.0414081805923563,
-0.00374633773382311));
#44591=CARTESIAN_POINT('Ctrl Pts',(-0.0161999999987847,-0.0413581243643992,
-0.00381889960619159));
#44592=CARTESIAN_POINT('Ctrl Pts',(-0.0159628235627429,-0.0414384247160303,
-0.00321302972381512));
#44593=CARTESIAN_POINT('Ctrl Pts',(-0.0160086241939108,-0.0414079981827581,
-0.00325294897397118));
#44594=CARTESIAN_POINT('Ctrl Pts',(-0.0160934832388146,-0.0413367207429093,
-0.00334646106679692));
#44595=CARTESIAN_POINT('Ctrl Pts',(-0.0161814674256218,-0.0412396136184735,
-0.00353217877322852));
#44596=CARTESIAN_POINT('Ctrl Pts',(-0.0162000031195221,-0.0411993385669745,
-0.00366927823060111));
#44597=CARTESIAN_POINT('Ctrl Pts',(-0.0161999999992124,-0.041175178948727,
-0.00374311636262439));
#44598=CARTESIAN_POINT('Ctrl Pts',(-0.0159803330326856,-0.0411244170199117,
-0.00319552025387248));
#44599=CARTESIAN_POINT('Ctrl Pts',(-0.0160240415983997,-0.0411163328788775,
-0.00323922980950275));
#44600=CARTESIAN_POINT('Ctrl Pts',(-0.0161023983074396,-0.0410987223439351,
-0.00333924835453889));
#44601=CARTESIAN_POINT('Ctrl Pts',(-0.0161808546695484,-0.0410703444398291,
-0.00352111890571466));
#44602=CARTESIAN_POINT('Ctrl Pts',(-0.0162000032226064,-0.0410527962950976,
-0.0036567880655664));
#44603=CARTESIAN_POINT('Ctrl Pts',(-0.0161999999991864,-0.0410443012976303,
-0.0037258852675939));
#44604=CARTESIAN_POINT('Ctrl Pts',(-0.0159803300851459,-0.0409788141462715,
-0.00319552320141217));
#44605=CARTESIAN_POINT('Ctrl Pts',(-0.0160266114141903,-0.0409788182295164,
-0.00324180453020668));
#44606=CARTESIAN_POINT('Ctrl Pts',(-0.0161069828280333,-0.0409788271246906,
-0.00334654796809965));
#44607=CARTESIAN_POINT('Ctrl Pts',(-0.0161827725636961,-0.0409788414577657,
-0.00352952438408725));
#44608=CARTESIAN_POINT('Ctrl Pts',(-0.0162000028998045,-0.0409788503201197,
-0.00366042730492668));
#44609=CARTESIAN_POINT('Ctrl Pts',(-0.0161999999992679,-0.0409788546105534,
-0.00372588633138973));
#44610=CARTESIAN_POINT('',(-0.0159803300858899,-0.040978887648424,-0.0031955232006682));
#44611=CARTESIAN_POINT('Ctrl Pts',(-0.0157883689863059,-0.0420671433761781,
-0.00338748430025228));
#44612=CARTESIAN_POINT('Ctrl Pts',(-0.0158238948255348,-0.0419960916977202,
-0.00335195846102329));
#44613=CARTESIAN_POINT('Ctrl Pts',(-0.0158828523983345,-0.0418424076018102,
-0.00329300088822358));
#44614=CARTESIAN_POINT('Ctrl Pts',(-0.0159628190767039,-0.0414384473777965,
-0.00321303420985414));
#44615=CARTESIAN_POINT('Ctrl Pts',(-0.0159803300858999,-0.0411244698616723,
-0.0031955232006582));
#44616=CARTESIAN_POINT('Ctrl Pts',(-0.0159803300858999,-0.040978887648414,
-0.0031955232006582));
#44617=CARTESIAN_POINT('',(-0.0162,-0.040978887648424,-0.00372585328655811));
#44618=CARTESIAN_POINT('Origin',(-0.01545000000001,-0.040978887648414,-0.00372585328654811));
#44619=CARTESIAN_POINT('Origin',(-0.01620000000001,-0.040978887648414,-0.00447574002801644));
#44620=CARTESIAN_POINT('Ctrl Pts',(-0.0157883510491122,-0.0420671792490158,
-0.00338750223744593));
#44621=CARTESIAN_POINT('Ctrl Pts',(-0.0158238849031059,-0.0419961175614541,
-0.0033519683834522));
#44622=CARTESIAN_POINT('Ctrl Pts',(-0.0158828479122755,-0.0418424302635563,
-0.00329300537428259));
#44623=CARTESIAN_POINT('Ctrl Pts',(-0.0159628235627429,-0.0414384247160304,
-0.00321302972381513));
#44624=CARTESIAN_POINT('Ctrl Pts',(-0.0159803330326856,-0.0411244170199117,
-0.00319552025387248));
#44625=CARTESIAN_POINT('Ctrl Pts',(-0.0159803300851459,-0.0409788141462716,
-0.00319552320141217));
#44626=CARTESIAN_POINT('Ctrl Pts',(-0.0157528254319766,-0.0420316530974381,
-0.00331644688517704));
#44627=CARTESIAN_POINT('Ctrl Pts',(-0.0157879192374373,-0.0419612102583594,
-0.00328819106591946));
#44628=CARTESIAN_POINT('Ctrl Pts',(-0.0158470801331243,-0.041807594796958,
-0.00323945968618903));
#44629=CARTESIAN_POINT('Ctrl Pts',(-0.015922904312587,-0.0414079981827581,
-0.00316722909264728));
#44630=CARTESIAN_POINT('Ctrl Pts',(-0.0159366234770553,-0.0411163328788775,
-0.00315181168815843));
#44631=CARTESIAN_POINT('Ctrl Pts',(-0.0159340487563514,-0.0409788182295164,
-0.00314924187236774));
#44632=CARTESIAN_POINT('Ctrl Pts',(-0.0156743980241011,-0.0419532255098914,
-0.00319535545324794));
#44633=CARTESIAN_POINT('Ctrl Pts',(-0.0157091531723962,-0.0418828002313692,
-0.00317674165713853));
#44634=CARTESIAN_POINT('Ctrl Pts',(-0.0157672464104804,-0.0417253071758865,
-0.0031410829300009));
#44635=CARTESIAN_POINT('Ctrl Pts',(-0.0158293922197611,-0.0413367207429093,
-0.00308237004774348));
#44636=CARTESIAN_POINT('Ctrl Pts',(-0.0158366049320192,-0.0410987223439351,
-0.00307345497911859));
#44637=CARTESIAN_POINT('Ctrl Pts',(-0.0158293053184584,-0.0409788271246907,
-0.00306887045852474));
#44638=CARTESIAN_POINT('Ctrl Pts',(-0.0154683058786476,-0.0417471348922467,
-0.00302722105556352));
#44639=CARTESIAN_POINT('Ctrl Pts',(-0.0155066139651694,-0.0416772361088086,
-0.00302017623900574));
#44640=CARTESIAN_POINT('Ctrl Pts',(-0.0155701075544912,-0.0415180843704948,
-0.00300445165805715));
#44641=CARTESIAN_POINT('Ctrl Pts',(-0.0156436745133296,-0.0412396136184735,
-0.00299438586093631));
#44642=CARTESIAN_POINT('Ctrl Pts',(-0.0156547343808434,-0.0410703444398291,
-0.00299499861700969));
#44643=CARTESIAN_POINT('Ctrl Pts',(-0.0156463289024708,-0.0409788414577657,
-0.002993080722862));
#44644=CARTESIAN_POINT('Ctrl Pts',(-0.0153031099239451,-0.0415819348578541,
-0.00297584464036246));
#44645=CARTESIAN_POINT('Ctrl Pts',(-0.0153491317045492,-0.041527830927245,
-0.00297584582608801));
#44646=CARTESIAN_POINT('Ctrl Pts',(-0.015429515552735,-0.0414081805923563,
-0.00297584847269227));
#44647=CARTESIAN_POINT('Ctrl Pts',(-0.0155065750559569,-0.0411993385669745,
-0.00297585016703602));
#44648=CARTESIAN_POINT('Ctrl Pts',(-0.0155190652209917,-0.0410527962950977,
-0.00297585006395169));
#44649=CARTESIAN_POINT('Ctrl Pts',(-0.0155154259816315,-0.0409788503201198,
-0.00297585038675357));
#44650=CARTESIAN_POINT('Ctrl Pts',(-0.0152303031410779,-0.0415091242546894,
-0.00297585328874096));
#44651=CARTESIAN_POINT('Ctrl Pts',(-0.0152765861541394,-0.0414628494275772,
-0.00297585328844161));
#44652=CARTESIAN_POINT('Ctrl Pts',(-0.0153569536803665,-0.0413581243643992,
-0.00297585328777345));
#44653=CARTESIAN_POINT('Ctrl Pts',(-0.0154327369239338,-0.041175178948727,
-0.00297585328734569));
#44654=CARTESIAN_POINT('Ctrl Pts',(-0.0154499680189642,-0.0410443012976304,
-0.00297585328737171));
#44655=CARTESIAN_POINT('Ctrl Pts',(-0.0154499669551684,-0.0409788546105535,
-0.00297585328729021));
#44656=CARTESIAN_POINT('',(-0.0152303632585517,-0.041509137648424,-0.00297585328655811));
#44657=CARTESIAN_POINT('Ctrl Pts',(-0.0157883689863059,-0.0420671433761781,
-0.00338748430025228));
#44658=CARTESIAN_POINT('Ctrl Pts',(-0.0157528431470768,-0.0420316175369492,
-0.00331643262179432));
#44659=CARTESIAN_POINT('Ctrl Pts',(-0.0156744155682287,-0.041953189958101,
-0.00319534605695119));
#44660=CARTESIAN_POINT('Ctrl Pts',(-0.0154683367770566,-0.0417471111669288,
-0.00302722693053075));
#44661=CARTESIAN_POINT('Ctrl Pts',(-0.0153031609543063,-0.0415819353441786,
-0.00297585328654811));
#44662=CARTESIAN_POINT('Ctrl Pts',(-0.0152303632585616,-0.041509137648434,
-0.00297585328654811));
#44663=CARTESIAN_POINT('',(-0.01545,-0.040978887648424,-0.00297585328655811));
#44664=CARTESIAN_POINT('Origin',(-0.0147001132585417,-0.040978887648414,
-0.00297585328654811));
#44665=CARTESIAN_POINT('Origin',(-0.01545000000001,-0.040978887648414,-0.00372585328654811));
#44666=CARTESIAN_POINT('Ctrl Pts',(0.00878840485914476,-0.0420671254389838,
-0.00338750223744656));
#44667=CARTESIAN_POINT('Ctrl Pts',(0.00871734317158273,-0.0421026592929779,
-0.00335196838345255));
#44668=CARTESIAN_POINT('Ctrl Pts',(0.00856365587368485,-0.0421616223021476,
-0.00329300537428275));
#44669=CARTESIAN_POINT('Ctrl Pts',(0.00815965032615725,-0.0422415979526155,
-0.00321302972381497));
#44670=CARTESIAN_POINT('Ctrl Pts',(0.00784564263003751,-0.042259107422558,
-0.00319552025387238));
#44671=CARTESIAN_POINT('Ctrl Pts',(0.00770003975639664,-0.0422591044750182,
-0.00319552320141217));
#44672=CARTESIAN_POINT('Ctrl Pts',(0.00875287870756702,-0.0420315998218482,
-0.00331644688517755));
#44673=CARTESIAN_POINT('Ctrl Pts',(0.00868243586848799,-0.0420666936273092,
-0.00328819106591975));
#44674=CARTESIAN_POINT('Ctrl Pts',(0.00852882040708653,-0.0421258545229965,
-0.00323945968618918));
#44675=CARTESIAN_POINT('Ctrl Pts',(0.00812922379288497,-0.0422016787024594,
-0.00316722909264713));
#44676=CARTESIAN_POINT('Ctrl Pts',(0.00783755848900357,-0.0422153978669278,
-0.00315181168815834));
#44677=CARTESIAN_POINT('Ctrl Pts',(0.00770004383964167,-0.0422128231462237,
-0.0031492418723677));
#44678=CARTESIAN_POINT('Ctrl Pts',(0.00867445112002032,-0.0419531724139727,
-0.00319535545324827));
#44679=CARTESIAN_POINT('Ctrl Pts',(0.00860402584149779,-0.041987927562268,
-0.00317674165713874));
#44680=CARTESIAN_POINT('Ctrl Pts',(0.00844653278601498,-0.0420460208003524,
-0.00314108293000102));
#44681=CARTESIAN_POINT('Ctrl Pts',(0.00805794635303622,-0.0421081666096336,
-0.00308237004774336));
#44682=CARTESIAN_POINT('Ctrl Pts',(0.00781994795406137,-0.0421153793218916,
-0.00307345497911853));
#44683=CARTESIAN_POINT('Ctrl Pts',(0.00770005273481621,-0.0421080797083306,
-0.00306887045852466));
#44684=CARTESIAN_POINT('Ctrl Pts',(0.00846836050237675,-0.0417470802685202,
-0.0030272210555645));
#44685=CARTESIAN_POINT('Ctrl Pts',(0.0083984617189383,-0.0417853883550424,
-0.00302017623900663));
#44686=CARTESIAN_POINT('Ctrl Pts',(0.00823930998062413,-0.0418488819443643,
-0.00300445165805787));
#44687=CARTESIAN_POINT('Ctrl Pts',(0.00796083922860127,-0.041922448903203,
-0.00299438586093674));
#44688=CARTESIAN_POINT('Ctrl Pts',(0.00779157004995592,-0.0419335087707168,
-0.00299499861701009));
#44689=CARTESIAN_POINT('Ctrl Pts',(0.0077000670678918,-0.041925103292344,
-0.00299308072286236));
#44690=CARTESIAN_POINT('Ctrl Pts',(0.00830316046798526,-0.0415818843138191,
-0.00297584464036324));
#44691=CARTESIAN_POINT('Ctrl Pts',(0.00824905653737577,-0.0416279060944235,
-0.00297584582608869));
#44692=CARTESIAN_POINT('Ctrl Pts',(0.008129406202486,-0.0417082899426093,
-0.00297584847269271));
#44693=CARTESIAN_POINT('Ctrl Pts',(0.00792056417710238,-0.0417853494458315,
-0.00297585016703631));
#44694=CARTESIAN_POINT('Ctrl Pts',(0.00777402190522474,-0.0417978396108661,
-0.00297585006395198));
#44695=CARTESIAN_POINT('Ctrl Pts',(0.00770007593024611,-0.0417942003715057,
-0.00297585038675383));
#44696=CARTESIAN_POINT('Ctrl Pts',(0.00823034986482126,-0.0415090775309527,
-0.00297585328874096));
#44697=CARTESIAN_POINT('Ctrl Pts',(0.00818407503770855,-0.0415553605440146,
-0.00297585328844161));
#44698=CARTESIAN_POINT('Ctrl Pts',(0.0080793499745296,-0.041635728070242,
-0.00297585328777345));
#44699=CARTESIAN_POINT('Ctrl Pts',(0.00789640455885557,-0.0417115113138095,
-0.00297585328734569));
#44700=CARTESIAN_POINT('Ctrl Pts',(0.00776552690775766,-0.0417287424088398,
-0.00297585328737171));
#44701=CARTESIAN_POINT('Ctrl Pts',(0.00770008022067996,-0.0417287413450437,
-0.00297585328729021));
#44702=CARTESIAN_POINT('',(0.0087883689862958,-0.0420671433761681,-0.00338748430026228));
#44703=CARTESIAN_POINT('',(0.0077001132585517,-0.0422591044757622,-0.0031955232006682));
#44704=CARTESIAN_POINT('Ctrl Pts',(0.0087883689863058,-0.0420671433761781,
-0.00338748430025228));
#44705=CARTESIAN_POINT('Ctrl Pts',(0.0087173173078479,-0.0421026692154071,
-0.00335195846102329));
#44706=CARTESIAN_POINT('Ctrl Pts',(0.0085636332119379,-0.0421616267882068,
-0.00329300088822358));
#44707=CARTESIAN_POINT('Ctrl Pts',(0.0081596729879242,-0.0422415934665763,
-0.00321303420985414));
#44708=CARTESIAN_POINT('Ctrl Pts',(0.00784569547182,-0.0422591044757722,
-0.0031955232006582));
#44709=CARTESIAN_POINT('Ctrl Pts',(0.0077001132585617,-0.0422591044757722,
-0.0031955232006582));
#44710=CARTESIAN_POINT('',(0.0082303632585517,-0.041509137648424,-0.00297585328655811));
#44711=CARTESIAN_POINT('Ctrl Pts',(0.0087883689863058,-0.0420671433761781,
-0.00338748430025228));
#44712=CARTESIAN_POINT('Ctrl Pts',(0.0087528431470769,-0.0420316175369492,
-0.00331643262179432));
#44713=CARTESIAN_POINT('Ctrl Pts',(0.0086744155682287,-0.041953189958101,
-0.00319534605695119));
#44714=CARTESIAN_POINT('Ctrl Pts',(0.0084683367770566,-0.0417471111669288,
-0.00302722693053075));
#44715=CARTESIAN_POINT('Ctrl Pts',(0.0083031609543063,-0.0415819353441786,
-0.00297585328654811));
#44716=CARTESIAN_POINT('Ctrl Pts',(0.0082303632585617,-0.041509137648434,
-0.00297585328654811));
#44717=CARTESIAN_POINT('',(0.0077001132585517,-0.0417287743898723,-0.00297585328655811));
#44718=CARTESIAN_POINT('Origin',(0.0077001132585617,-0.040978887648414,
-0.00297585328654811));
#44719=CARTESIAN_POINT('Origin',(0.0077001132585617,-0.0417287743898823,
-0.00372585328654811));
#44720=CARTESIAN_POINT('Ctrl Pts',(0.00878835104911207,-0.042067179249016,
-0.00338750223744602));
#44721=CARTESIAN_POINT('Ctrl Pts',(0.00875282543197647,-0.0420316530974382,
-0.00331644688517711));
#44722=CARTESIAN_POINT('Ctrl Pts',(0.00867439802410098,-0.0419532255098915,
-0.00319535545324799));
#44723=CARTESIAN_POINT('Ctrl Pts',(0.00846830587865056,-0.04174713489225,
-0.00302722105556606));
#44724=CARTESIAN_POINT('Ctrl Pts',(0.00830310992395243,-0.0415819348578616,
-0.00297584464036477));
#44725=CARTESIAN_POINT('Ctrl Pts',(0.00823030314108757,-0.0415091242546993,
-0.00297585328874096));
#44726=CARTESIAN_POINT('Ctrl Pts',(0.00882388490310585,-0.0419961175614542,
-0.00335196838345225));
#44727=CARTESIAN_POINT('Ctrl Pts',(0.00878791923743725,-0.0419612102583595,
-0.0032881910659195));
#44728=CARTESIAN_POINT('Ctrl Pts',(0.00870915317239613,-0.0418828002313693,
-0.00317674165713856));
#44729=CARTESIAN_POINT('Ctrl Pts',(0.0085066139651724,-0.0416772361088118,
-0.0030201762390081));
#44730=CARTESIAN_POINT('Ctrl Pts',(0.00834913170455625,-0.0415278309272518,
-0.00297584582609));
#44731=CARTESIAN_POINT('Ctrl Pts',(0.00827658615414919,-0.0414628494275861,
-0.00297585328844161));
#44732=CARTESIAN_POINT('Ctrl Pts',(0.00888284791227546,-0.0418424302635565,
-0.00329300537428262));
#44733=CARTESIAN_POINT('Ctrl Pts',(0.00884708013312432,-0.0418075947969581,
-0.00323945968618904));
#44734=CARTESIAN_POINT('Ctrl Pts',(0.00876724641048024,-0.0417253071758866,
-0.00314108293000092));
#44735=CARTESIAN_POINT('Ctrl Pts',(0.00857010755449411,-0.041518084370498,
-0.0030044516580592));
#44736=CARTESIAN_POINT('Ctrl Pts',(0.00842951555274125,-0.0414081805923613,
-0.00297584847269355));
#44737=CARTESIAN_POINT('Ctrl Pts',(0.0083569536803763,-0.041358124364406,
-0.00297585328777345));
#44738=CARTESIAN_POINT('Ctrl Pts',(0.00896282356274304,-0.0414384247160302,
-0.0032130297238151));
#44739=CARTESIAN_POINT('Ctrl Pts',(0.00892290431258698,-0.041407998182758,
-0.00316722909264726));
#44740=CARTESIAN_POINT('Ctrl Pts',(0.00882939221976126,-0.0413367207429092,
-0.00308237004774346));
#44741=CARTESIAN_POINT('Ctrl Pts',(0.00864367451333237,-0.0412396136184749,
-0.00299438586093763));
#44742=CARTESIAN_POINT('Ctrl Pts',(0.00850657505596322,-0.0411993385669762,
-0.00297585016703686));
#44743=CARTESIAN_POINT('Ctrl Pts',(0.00843273692394366,-0.0411751789487302,
-0.00297585328734569));
#44744=CARTESIAN_POINT('Ctrl Pts',(0.00898033303268563,-0.0411244170199114,
-0.00319552025387247));
#44745=CARTESIAN_POINT('Ctrl Pts',(0.00893662347705534,-0.0411163328788773,
-0.00315181168815842));
#44746=CARTESIAN_POINT('Ctrl Pts',(0.00883660493201919,-0.0410987223439349,
-0.00307345497911858));
#44747=CARTESIAN_POINT('Ctrl Pts',(0.00865473438084623,-0.0410703444398294,
-0.00299499861701086));
#44748=CARTESIAN_POINT('Ctrl Pts',(0.00851906522099781,-0.0410527962950983,
-0.00297585006395255));
#44749=CARTESIAN_POINT('Ctrl Pts',(0.00844996801897355,-0.0410443012976314,
-0.00297585328737171));
#44750=CARTESIAN_POINT('Ctrl Pts',(0.00898033008514593,-0.0409788141462712,
-0.00319552320141217));
#44751=CARTESIAN_POINT('Ctrl Pts',(0.00893404875635143,-0.0409788182295161,
-0.00314924187236774));
#44752=CARTESIAN_POINT('Ctrl Pts',(0.00882930531845842,-0.0409788271246904,
-0.00306887045852473));
#44753=CARTESIAN_POINT('Ctrl Pts',(0.00864632890247355,-0.0409788414577655,
-0.00299308072286314));
#44754=CARTESIAN_POINT('Ctrl Pts',(0.00851542598163733,-0.0409788503201196,
-0.00297585038675435));
#44755=CARTESIAN_POINT('Ctrl Pts',(0.00844996695517721,-0.0409788546105533,
-0.00297585328729021));
#44756=CARTESIAN_POINT('',(0.0089803300858899,-0.040978887648424,-0.0031955232006682));
#44757=CARTESIAN_POINT('Ctrl Pts',(0.0087883689863058,-0.0420671433761781,
-0.00338748430025228));
#44758=CARTESIAN_POINT('Ctrl Pts',(0.0088238948255348,-0.0419960916977202,
-0.00335195846102329));
#44759=CARTESIAN_POINT('Ctrl Pts',(0.0088828523983345,-0.0418424076018102,
-0.00329300088822358));
#44760=CARTESIAN_POINT('Ctrl Pts',(0.008962819076704,-0.0414384473777965,
-0.00321303420985414));
#44761=CARTESIAN_POINT('Ctrl Pts',(0.0089803300858999,-0.0411244698616723,
-0.0031955232006582));
#44762=CARTESIAN_POINT('Ctrl Pts',(0.0089803300858999,-0.040978887648414,
-0.0031955232006582));
#44763=CARTESIAN_POINT('',(0.00845,-0.040978887648424,-0.00297585328655811));
#44764=CARTESIAN_POINT('Origin',(0.00845000000001,-0.040978887648414,-0.00372585328654811));
#44765=CARTESIAN_POINT('Origin',(0.0077001132585617,-0.040978887648414,
-0.00297585328654811));
#44766=CARTESIAN_POINT('Ctrl Pts',(0.00878835104911214,-0.0420671792490158,
-0.00338750223744593));
#44767=CARTESIAN_POINT('Ctrl Pts',(0.00882388490310589,-0.0419961175614541,
-0.0033519683834522));
#44768=CARTESIAN_POINT('Ctrl Pts',(0.00888284791227549,-0.0418424302635564,
-0.0032930053742826));
#44769=CARTESIAN_POINT('Ctrl Pts',(0.00896282356274302,-0.0414384247160304,
-0.00321302972381512));
#44770=CARTESIAN_POINT('Ctrl Pts',(0.00898033303268562,-0.0411244170199117,
-0.00319552025387248));
#44771=CARTESIAN_POINT('Ctrl Pts',(0.00898033008514593,-0.0409788141462715,
-0.00319552320141217));
#44772=CARTESIAN_POINT('Ctrl Pts',(0.00885940640138106,-0.0420316530974381,
-0.00342302785458162));
#44773=CARTESIAN_POINT('Ctrl Pts',(0.00888766222063862,-0.0419612102583594,
-0.00338793404912082));
#44774=CARTESIAN_POINT('Ctrl Pts',(0.00893639360036903,-0.041807594796958,
-0.00332877315343381));
#44775=CARTESIAN_POINT('Ctrl Pts',(0.00900862419391088,-0.0414079981827581,
-0.00325294897397118));
#44776=CARTESIAN_POINT('Ctrl Pts',(0.00902404159839969,-0.0411163328788775,
-0.00323922980950275));
#44777=CARTESIAN_POINT('Ctrl Pts',(0.00902661141419034,-0.0409788182295164,
-0.00324180453020668));
#44778=CARTESIAN_POINT('Ctrl Pts',(0.00898049783331014,-0.0419532255098914,
-0.00350145526245707));
#44779=CARTESIAN_POINT('Ctrl Pts',(0.00899911162941954,-0.0418828002313692,
-0.00346670011416197));
#44780=CARTESIAN_POINT('Ctrl Pts',(0.00903477035655726,-0.0417253071758865,
-0.0034086068760778));
#44781=CARTESIAN_POINT('Ctrl Pts',(0.00909348323881464,-0.0413367207429093,
-0.00334646106679692));
#44782=CARTESIAN_POINT('Ctrl Pts',(0.00910239830743949,-0.0410987223439351,
-0.00333924835453889));
#44783=CARTESIAN_POINT('Ctrl Pts',(0.00910698282803342,-0.0409788271246906,
-0.00334654796809965));
#44784=CARTESIAN_POINT('Ctrl Pts',(0.00914863223099463,-0.0417471348922468,
-0.00370754740791059));
#44785=CARTESIAN_POINT('Ctrl Pts',(0.00915567704755241,-0.0416772361088086,
-0.0036692393213887));
#44786=CARTESIAN_POINT('Ctrl Pts',(0.00917140162850093,-0.0415180843704948,
-0.0036057457320669));
#44787=CARTESIAN_POINT('Ctrl Pts',(0.00918146742562174,-0.0412396136184735,
-0.00353217877322852));
#44788=CARTESIAN_POINT('Ctrl Pts',(0.00918085466954842,-0.0410703444398291,
-0.00352111890571465));
#44789=CARTESIAN_POINT('Ctrl Pts',(0.00918277256369609,-0.0409788414577657,
-0.00352952438408724));
#44790=CARTESIAN_POINT('Ctrl Pts',(0.00920000864619565,-0.0415819348578541,
-0.00387274336261302));
#44791=CARTESIAN_POINT('Ctrl Pts',(0.0092000074604701,-0.041527830927245,
-0.00382672158200887));
#44792=CARTESIAN_POINT('Ctrl Pts',(0.00920000481386584,-0.0414081805923563,
-0.00374633773382311));
#44793=CARTESIAN_POINT('Ctrl Pts',(0.00920000311952209,-0.0411993385669745,
-0.00366927823060111));
#44794=CARTESIAN_POINT('Ctrl Pts',(0.00920000322260642,-0.0410527962950976,
-0.0036567880655664));
#44795=CARTESIAN_POINT('Ctrl Pts',(0.00920000289980454,-0.0409788503201197,
-0.00366042730492667));
#44796=CARTESIAN_POINT('Ctrl Pts',(0.00919999999781715,-0.0415091242546894,
-0.00394555014548031));
#44797=CARTESIAN_POINT('Ctrl Pts',(0.0091999999981165,-0.0414628494275772,
-0.00389926713241869));
#44798=CARTESIAN_POINT('Ctrl Pts',(0.00919999999878466,-0.0413581243643992,
-0.00381889960619159));
#44799=CARTESIAN_POINT('Ctrl Pts',(0.00919999999921242,-0.041175178948727,
-0.00374311636262439));
#44800=CARTESIAN_POINT('Ctrl Pts',(0.0091999999991864,-0.0410443012976303,
-0.0037258852675939));
#44801=CARTESIAN_POINT('Ctrl Pts',(0.0091999999992679,-0.0409788546105534,
-0.00372588633138973));
#44802=CARTESIAN_POINT('',(0.0092,-0.041509137648424,-0.00394549002800645));
#44803=CARTESIAN_POINT('Ctrl Pts',(0.0087883689863058,-0.0420671433761781,
-0.00338748430025228));
#44804=CARTESIAN_POINT('Ctrl Pts',(0.0088594206647638,-0.0420316175369492,
-0.00342301013948126));
#44805=CARTESIAN_POINT('Ctrl Pts',(0.0089805072296069,-0.041953189958101,
-0.00350143771832943));
#44806=CARTESIAN_POINT('Ctrl Pts',(0.0091486263560274,-0.0417471111669288,
-0.00370751650950155));
#44807=CARTESIAN_POINT('Ctrl Pts',(0.00920000000001,-0.0415819353441786,
-0.00387269233225182));
#44808=CARTESIAN_POINT('Ctrl Pts',(0.00920000000001,-0.041509137648434,
-0.00394549002799644));
#44809=CARTESIAN_POINT('',(0.0092,-0.040978887648424,-0.00372585328655811));
#44810=CARTESIAN_POINT('Origin',(0.00920000000001,-0.040978887648414,-0.00447574002801644));
#44811=CARTESIAN_POINT('Origin',(0.00845000000001,-0.040978887648414,-0.00372585328654811));
#44812=CARTESIAN_POINT('Ctrl Pts',(0.00878835104911214,-0.0420671254389844,
-0.00338744842741457));
#44813=CARTESIAN_POINT('Ctrl Pts',(0.00885940640138106,-0.0420315998218488,
-0.00342297457899238));
#44814=CARTESIAN_POINT('Ctrl Pts',(0.00898049783331015,-0.0419531724139734,
-0.00350140216653905));
#44815=CARTESIAN_POINT('Ctrl Pts',(0.00914863223099464,-0.0417470802685199,
-0.00370749278418369));
#44816=CARTESIAN_POINT('Ctrl Pts',(0.00920000864619566,-0.0415818843138174,
-0.00387269281857635));
#44817=CARTESIAN_POINT('Ctrl Pts',(0.00919999999781715,-0.0415090775309502,
-0.00394550342174106));
#44818=CARTESIAN_POINT('Ctrl Pts',(0.00882388490310589,-0.0421026592929782,
-0.00345851011497631));
#44819=CARTESIAN_POINT('Ctrl Pts',(0.00888766222063861,-0.0420666936273096,
-0.003493417418071));
#44820=CARTESIAN_POINT('Ctrl Pts',(0.00899911162941954,-0.0419879275622684,
-0.00357182744506123));
#44821=CARTESIAN_POINT('Ctrl Pts',(0.00915567704755241,-0.0417853883550417,
-0.00377739156762174));
#44822=CARTESIAN_POINT('Ctrl Pts',(0.0092000074604701,-0.0416279060944215,
-0.00392679674918539));
#44823=CARTESIAN_POINT('Ctrl Pts',(0.0091999999981165,-0.0415553605440118,
-0.00399177824885322));
#44824=CARTESIAN_POINT('Ctrl Pts',(0.00888284791227548,-0.0421616223021478,
-0.00361219741287406));
#44825=CARTESIAN_POINT('Ctrl Pts',(0.00893639360036912,-0.0421258545229966,
-0.00364703287947235));
#44826=CARTESIAN_POINT('Ctrl Pts',(0.00903477035655715,-0.0420460208003526,
-0.00372932050054387));
#44827=CARTESIAN_POINT('Ctrl Pts',(0.00917140162850093,-0.0418488819443635,
-0.00393654330593559));
#44828=CARTESIAN_POINT('Ctrl Pts',(0.00920000481386584,-0.0417082899426073,
-0.00404644708407417));
#44829=CARTESIAN_POINT('Ctrl Pts',(0.00919999999878465,-0.0416357280702388,
-0.00409650331203123));
#44830=CARTESIAN_POINT('Ctrl Pts',(0.00896282356274302,-0.0422415979526153,
-0.00401620296040005));
#44831=CARTESIAN_POINT('Ctrl Pts',(0.00900862419391088,-0.0422016787024593,
-0.00404662949367235));
#44832=CARTESIAN_POINT('Ctrl Pts',(0.00909348323881464,-0.0421081666096335,
-0.00411790693352111));
#44833=CARTESIAN_POINT('Ctrl Pts',(0.00918146742562184,-0.0419224489032019,
-0.00421501405795684));
#44834=CARTESIAN_POINT('Ctrl Pts',(0.00920000311952209,-0.0417853494458292,
-0.00425528910945596));
#44835=CARTESIAN_POINT('Ctrl Pts',(0.00919999999921242,-0.041711511313806,
-0.00427944872770334));
#44836=CARTESIAN_POINT('Ctrl Pts',(0.00898033303268561,-0.0422591074225579,
-0.00433021065651873));
#44837=CARTESIAN_POINT('Ctrl Pts',(0.00902404159839969,-0.0422153978669277,
-0.00433829479755288));
#44838=CARTESIAN_POINT('Ctrl Pts',(0.00910239830743949,-0.0421153793218916,
-0.00435590533249531));
#44839=CARTESIAN_POINT('Ctrl Pts',(0.00918085466954842,-0.0419335087707158,
-0.00438428323660133));
#44840=CARTESIAN_POINT('Ctrl Pts',(0.00920000322260641,-0.041797839610864,
-0.00440183138133278));
#44841=CARTESIAN_POINT('Ctrl Pts',(0.0091999999991864,-0.0417287424088365,
-0.00441032637880008));
#44842=CARTESIAN_POINT('Ctrl Pts',(0.00898033008514593,-0.0422591044750182,
-0.00447581353015895));
#44843=CARTESIAN_POINT('Ctrl Pts',(0.00902661141419034,-0.0422128231462237,
-0.00447580944691406));
#44844=CARTESIAN_POINT('Ctrl Pts',(0.00910698282803332,-0.0421080797083307,
-0.00447580055173983));
#44845=CARTESIAN_POINT('Ctrl Pts',(0.00918277256369609,-0.0419251032923432,
-0.00447578621866474));
#44846=CARTESIAN_POINT('Ctrl Pts',(0.00920000289980454,-0.0417942003715037,
-0.00447577735631073));
#44847=CARTESIAN_POINT('Ctrl Pts',(0.0091999999992679,-0.0417287413450407,
-0.00447577306587704));
#44848=CARTESIAN_POINT('',(0.0089803300858899,-0.0422591044757622,-0.00447574002800645));
#44849=CARTESIAN_POINT('Ctrl Pts',(0.0087883689863058,-0.0420671433761781,
-0.00338748430025228));
#44850=CARTESIAN_POINT('Ctrl Pts',(0.0088238948255348,-0.0421026692154071,
-0.00345853597871023));
#44851=CARTESIAN_POINT('Ctrl Pts',(0.0088828523983345,-0.0421616267882069,
-0.00361222007462022));
#44852=CARTESIAN_POINT('Ctrl Pts',(0.008962819076704,-0.0422415934665763,
-0.00401618029863389));
#44853=CARTESIAN_POINT('Ctrl Pts',(0.0089803300858999,-0.0422591044757722,
-0.00433015781475808));
#44854=CARTESIAN_POINT('Ctrl Pts',(0.0089803300858999,-0.0422591044757722,
-0.00447574002801644));
#44855=CARTESIAN_POINT('',(0.0092,-0.0417287743898723,-0.00447574002800645));
#44856=CARTESIAN_POINT('Origin',(0.00845000000001,-0.0417287743898823,-0.00447574002801644));
#44857=CARTESIAN_POINT('Origin',(0.00920000000001,-0.040978887648414,-0.00447574002801644));
#44858=CARTESIAN_POINT('Ctrl Pts',(0.00878835104911207,-0.0420671254389844,
-0.00338744842741442));
#44859=CARTESIAN_POINT('Ctrl Pts',(0.00882388490310585,-0.0421026592929781,
-0.00345851011497621));
#44860=CARTESIAN_POINT('Ctrl Pts',(0.00888284791227546,-0.0421616223021478,
-0.00361219741287397));
#44861=CARTESIAN_POINT('Ctrl Pts',(0.00896282356274304,-0.0422415979526153,
-0.00401620296040014));
#44862=CARTESIAN_POINT('Ctrl Pts',(0.00898033303268563,-0.0422591074225579,
-0.00433021065651894));
#44863=CARTESIAN_POINT('Ctrl Pts',(0.00898033008514593,-0.0422591044750182,
-0.00447581353015925));
#44864=CARTESIAN_POINT('Ctrl Pts',(0.00875282543197647,-0.0421381807912533,
-0.00342297457899223));
#44865=CARTESIAN_POINT('Ctrl Pts',(0.00878791923743725,-0.0421664366105109,
-0.00349341741807089));
#44866=CARTESIAN_POINT('Ctrl Pts',(0.00884708013312432,-0.0422151679902414,
-0.00364703287947226));
#44867=CARTESIAN_POINT('Ctrl Pts',(0.00892290431258698,-0.0422873985837832,
-0.00404662949367244));
#44868=CARTESIAN_POINT('Ctrl Pts',(0.00893662347705534,-0.042302815988272,
-0.00433829479755307));
#44869=CARTESIAN_POINT('Ctrl Pts',(0.00893404875635143,-0.0423053858040627,
-0.00447580944691434));
#44870=CARTESIAN_POINT('Ctrl Pts',(0.00867439802410098,-0.0422592722231824,
-0.00350140216653891));
#44871=CARTESIAN_POINT('Ctrl Pts',(0.00870915317239614,-0.0422778860192918,
-0.00357182744506112));
#44872=CARTESIAN_POINT('Ctrl Pts',(0.00876724641048024,-0.0423135447464296,
-0.00372932050054379));
#44873=CARTESIAN_POINT('Ctrl Pts',(0.00882939221976126,-0.042372257628687,
-0.00411790693352119));
#44874=CARTESIAN_POINT('Ctrl Pts',(0.00883660493201919,-0.0423811726973118,
-0.00435590533249547));
#44875=CARTESIAN_POINT('Ctrl Pts',(0.00882930531845843,-0.0423857572179057,
-0.00447580055174007));
#44876=CARTESIAN_POINT('Ctrl Pts',(0.00846830587865057,-0.0424274066208644,
-0.00370749278418045));
#44877=CARTESIAN_POINT('Ctrl Pts',(0.00850661396517241,-0.0424344514374222,
-0.00377739156761855));
#44878=CARTESIAN_POINT('Ctrl Pts',(0.00857010755449421,-0.0424501760183713,
-0.00393654330593241));
#44879=CARTESIAN_POINT('Ctrl Pts',(0.00864367451333238,-0.0424602418154928,
-0.00421501405795545));
#44880=CARTESIAN_POINT('Ctrl Pts',(0.00865473438084623,-0.0424596290594195,
-0.00438428323660103));
#44881=CARTESIAN_POINT('Ctrl Pts',(0.00864632890247365,-0.0424615469535673,
-0.00447578621866493));
#44882=CARTESIAN_POINT('Ctrl Pts',(0.00830310992395244,-0.0424787830360656,
-0.00387269281856879));
#44883=CARTESIAN_POINT('Ctrl Pts',(0.00834913170455626,-0.0424787818503404,
-0.00392679674917857));
#44884=CARTESIAN_POINT('Ctrl Pts',(0.00842951555274136,-0.0424787792037368,
-0.00404644708406916));
#44885=CARTESIAN_POINT('Ctrl Pts',(0.00850657505596322,-0.0424787775093936,
-0.0042552891094542));
#44886=CARTESIAN_POINT('Ctrl Pts',(0.00851906522099781,-0.0424787776124778,
-0.00440183138133209));
#44887=CARTESIAN_POINT('Ctrl Pts',(0.00851542598163734,-0.0424787772896761,
-0.00447577735631089));
#44888=CARTESIAN_POINT('Ctrl Pts',(0.00823030314108758,-0.0424787743876895,
-0.00394550342173112));
#44889=CARTESIAN_POINT('Ctrl Pts',(0.0082765861541492,-0.0424787743879888,
-0.00399177824884436));
#44890=CARTESIAN_POINT('Ctrl Pts',(0.00835695368037631,-0.042478774388657,
-0.00409650331202441));
#44891=CARTESIAN_POINT('Ctrl Pts',(0.00843273692394367,-0.0424787743890847,
-0.00427944872770011));
#44892=CARTESIAN_POINT('Ctrl Pts',(0.00844996801897356,-0.0424787743890587,
-0.00441032637879902));
#44893=CARTESIAN_POINT('Ctrl Pts',(0.00844996695517722,-0.0424787743891402,
-0.00447577306587717));
#44894=CARTESIAN_POINT('',(0.0082303632585517,-0.0424787743898723,-0.00394549002800645));
#44895=CARTESIAN_POINT('Ctrl Pts',(0.0087883689863058,-0.0420671433761781,
-0.00338748430025228));
#44896=CARTESIAN_POINT('Ctrl Pts',(0.0087528431470769,-0.0421381950546361,
-0.00342301013948126));
#44897=CARTESIAN_POINT('Ctrl Pts',(0.0086744155682287,-0.0422592816194792,
-0.00350143771832943));
#44898=CARTESIAN_POINT('Ctrl Pts',(0.0084683367770566,-0.0424274007458997,
-0.00370751650950155));
#44899=CARTESIAN_POINT('Ctrl Pts',(0.0083031609543063,-0.0424787743898823,
-0.00387269233225182));
#44900=CARTESIAN_POINT('Ctrl Pts',(0.0082303632585617,-0.0424787743898823,
-0.00394549002799644));
#44901=CARTESIAN_POINT('',(0.00845,-0.0424787743898723,-0.00447574002800645));
#44902=CARTESIAN_POINT('Origin',(0.0077001132585617,-0.0424787743898823,
-0.00447574002801644));
#44903=CARTESIAN_POINT('Origin',(0.00845000000001,-0.0417287743898823,-0.00447574002801644));
#44904=CARTESIAN_POINT('Ctrl Pts',(-0.0157883510491121,-0.042067179249016,
-0.0209642043356702));
#44905=CARTESIAN_POINT('Ctrl Pts',(-0.0158238849031058,-0.0419961175614543,
-0.0209997381896639));
#44906=CARTESIAN_POINT('Ctrl Pts',(-0.0158828479122755,-0.0418424302635564,
-0.0210587011988336));
#44907=CARTESIAN_POINT('Ctrl Pts',(-0.0159628235627429,-0.0414384247160302,
-0.0211386768493011));
#44908=CARTESIAN_POINT('Ctrl Pts',(-0.0159803330326856,-0.0411244170199114,
-0.0211561863192437));
#44909=CARTESIAN_POINT('Ctrl Pts',(-0.0159803300851459,-0.0409788141462712,
-0.021156183371704));
#44910=CARTESIAN_POINT('Ctrl Pts',(-0.015859406401381,-0.0420316530974383,
-0.0209286787185346));
#44911=CARTESIAN_POINT('Ctrl Pts',(-0.0158876622206386,-0.0419612102583595,
-0.0209637725239953));
#44912=CARTESIAN_POINT('Ctrl Pts',(-0.0159363936003691,-0.0418075947969582,
-0.0210229334196824));
#44913=CARTESIAN_POINT('Ctrl Pts',(-0.0160086241939108,-0.041407998182758,
-0.0210987575991451));
#44914=CARTESIAN_POINT('Ctrl Pts',(-0.0160240415983997,-0.0411163328788773,
-0.0211124767636134));
#44915=CARTESIAN_POINT('Ctrl Pts',(-0.0160266114141903,-0.0409788182295161,
-0.0211099020429095));
#44916=CARTESIAN_POINT('Ctrl Pts',(-0.0159804978333101,-0.0419532255098915,
-0.0208502513106591));
#44917=CARTESIAN_POINT('Ctrl Pts',(-0.0159991116294195,-0.0418828002313693,
-0.0208850064589542));
#44918=CARTESIAN_POINT('Ctrl Pts',(-0.0160347703565571,-0.0417253071758866,
-0.0209430996970383));
#44919=CARTESIAN_POINT('Ctrl Pts',(-0.0160934832388147,-0.0413367207429092,
-0.0210052455063193));
#44920=CARTESIAN_POINT('Ctrl Pts',(-0.0161023983074396,-0.0410987223439349,
-0.0210124582185773));
#44921=CARTESIAN_POINT('Ctrl Pts',(-0.0161069828280333,-0.0409788271246903,
-0.0210051586050165));
#44922=CARTESIAN_POINT('Ctrl Pts',(-0.0161486322309921,-0.04174713489225,
-0.0206441591652087));
#44923=CARTESIAN_POINT('Ctrl Pts',(-0.0161556770475501,-0.0416772361088118,
-0.0206824672517305));
#44924=CARTESIAN_POINT('Ctrl Pts',(-0.0161714016284989,-0.041518084370498,
-0.0207459608410522));
#44925=CARTESIAN_POINT('Ctrl Pts',(-0.0161814674256205,-0.0412396136184749,
-0.0208195277998905));
#44926=CARTESIAN_POINT('Ctrl Pts',(-0.0161808546695472,-0.0410703444398294,
-0.0208305876674043));
#44927=CARTESIAN_POINT('Ctrl Pts',(-0.016182772563695,-0.0409788414577655,
-0.0208221821890317));
#44928=CARTESIAN_POINT('Ctrl Pts',(-0.0162000086461933,-0.0415819348578615,
-0.0204789632105105));
#44929=CARTESIAN_POINT('Ctrl Pts',(-0.0162000074604681,-0.0415278309272518,
-0.0205249849911143));
#44930=CARTESIAN_POINT('Ctrl Pts',(-0.0162000048138646,-0.0414081805923612,
-0.0206053688392993));
#44931=CARTESIAN_POINT('Ctrl Pts',(-0.0162000031195212,-0.0411993385669761,
-0.0206824283425213));
#44932=CARTESIAN_POINT('Ctrl Pts',(-0.0162000032226055,-0.0410527962950982,
-0.0206949185075559));
#44933=CARTESIAN_POINT('Ctrl Pts',(-0.0162000028998038,-0.0409788503201196,
-0.0206912792681954));
#44934=CARTESIAN_POINT('Ctrl Pts',(-0.0161999999978171,-0.0415091242546993,
-0.0204061564276456));
#44935=CARTESIAN_POINT('Ctrl Pts',(-0.0161999999981165,-0.0414628494275861,
-0.0204524394407073));
#44936=CARTESIAN_POINT('Ctrl Pts',(-0.0161999999987847,-0.041358124364406,
-0.0205328069669344));
#44937=CARTESIAN_POINT('Ctrl Pts',(-0.0161999999992124,-0.0411751789487302,
-0.0206085902105018));
#44938=CARTESIAN_POINT('Ctrl Pts',(-0.0161999999991864,-0.0410443012976313,
-0.0206258213055316));
#44939=CARTESIAN_POINT('Ctrl Pts',(-0.0161999999992679,-0.0409788546105533,
-0.0206258202417353));
#44940=CARTESIAN_POINT('',(-0.0157883689862958,-0.0420671433761681,-0.0209642222728539));
#44941=CARTESIAN_POINT('',(-0.0159803300858899,-0.040978887648424,-0.021156183372448));
#44942=CARTESIAN_POINT('Ctrl Pts',(-0.0157883689863059,-0.0420671433761781,
-0.0209642222728639));
#44943=CARTESIAN_POINT('Ctrl Pts',(-0.0158238948255348,-0.0419960916977202,
-0.0209997481120929));
#44944=CARTESIAN_POINT('Ctrl Pts',(-0.0158828523983345,-0.0418424076018101,
-0.0210587056848926));
#44945=CARTESIAN_POINT('Ctrl Pts',(-0.0159628190767039,-0.0414384473777965,
-0.0211386723632621));
#44946=CARTESIAN_POINT('Ctrl Pts',(-0.0159803300858999,-0.0411244698616723,
-0.021156183372458));
#44947=CARTESIAN_POINT('Ctrl Pts',(-0.0159803300858999,-0.040978887648414,
-0.021156183372458));
#44948=CARTESIAN_POINT('',(-0.0162,-0.041509137648424,-0.0204062165451098));
#44949=CARTESIAN_POINT('Ctrl Pts',(-0.0157883689863059,-0.0420671433761781,
-0.0209642222728639));
#44950=CARTESIAN_POINT('Ctrl Pts',(-0.0158594206647638,-0.0420316175369492,
-0.020928696433635));
#44951=CARTESIAN_POINT('Ctrl Pts',(-0.0159805072296069,-0.0419531899581009,
-0.0208502688547868));
#44952=CARTESIAN_POINT('Ctrl Pts',(-0.0161486263560273,-0.0417471111669288,
-0.0206441900636147));
#44953=CARTESIAN_POINT('Ctrl Pts',(-0.01620000000001,-0.0415819353441786,
-0.0204790142408644));
#44954=CARTESIAN_POINT('Ctrl Pts',(-0.01620000000001,-0.041509137648434,
-0.0204062165451198));
#44955=CARTESIAN_POINT('',(-0.0162,-0.040978887648424,-0.0206258532865581));
#44956=CARTESIAN_POINT('Origin',(-0.01620000000001,-0.040978887648414,-0.0198759665451198));
#44957=CARTESIAN_POINT('Origin',(-0.01545000000001,-0.040978887648414,-0.0206258532865681));
#44958=CARTESIAN_POINT('Ctrl Pts',(-0.0157883510491115,-0.0420671254389838,
-0.0209642581457029));
#44959=CARTESIAN_POINT('Ctrl Pts',(-0.0158594064013806,-0.0420315998218482,
-0.0209287319941251));
#44960=CARTESIAN_POINT('Ctrl Pts',(-0.0159804978333098,-0.0419531724139726,
-0.0208503044065784));
#44961=CARTESIAN_POINT('Ctrl Pts',(-0.0161486322309936,-0.0417470802685202,
-0.0206442137889348));
#44962=CARTESIAN_POINT('Ctrl Pts',(-0.0162000086461949,-0.041581884313819,
-0.0204790137545434));
#44963=CARTESIAN_POINT('Ctrl Pts',(-0.0161999999978171,-0.0415090775309527,
-0.0204062031513794));
#44964=CARTESIAN_POINT('Ctrl Pts',(-0.0158238849031055,-0.0421026592929779,
-0.0208931964581408));
#44965=CARTESIAN_POINT('Ctrl Pts',(-0.0158876622206383,-0.0420666936273093,
-0.0208582891550461));
#44966=CARTESIAN_POINT('Ctrl Pts',(-0.0159991116294193,-0.041987927562268,
-0.0207798791280559));
#44967=CARTESIAN_POINT('Ctrl Pts',(-0.0161556770475515,-0.0417853883550424,
-0.0205743150054964));
#44968=CARTESIAN_POINT('Ctrl Pts',(-0.0162000074604694,-0.0416279060944235,
-0.0204249098239339));
#44969=CARTESIAN_POINT('Ctrl Pts',(-0.0161999999981165,-0.0415553605440146,
-0.0203599283242667));
#44970=CARTESIAN_POINT('Ctrl Pts',(-0.0158828479122753,-0.0421616223021476,
-0.020739509160243));
#44971=CARTESIAN_POINT('Ctrl Pts',(-0.015936393600369,-0.0421258545229965,
-0.0207046736936446));
#44972=CARTESIAN_POINT('Ctrl Pts',(-0.016034770356557,-0.0420460208003524,
-0.0206223860725731));
#44973=CARTESIAN_POINT('Ctrl Pts',(-0.0161714016285002,-0.0418488819443643,
-0.0204151632671822));
#44974=CARTESIAN_POINT('Ctrl Pts',(-0.0162000048138654,-0.0417082899426093,
-0.0203052594890441));
#44975=CARTESIAN_POINT('Ctrl Pts',(-0.0161999999987847,-0.041635728070242,
-0.0202552032610877));
#44976=CARTESIAN_POINT('Ctrl Pts',(-0.0159628235627431,-0.0422415979526155,
-0.0203355036127153));
#44977=CARTESIAN_POINT('Ctrl Pts',(-0.0160086241939109,-0.0422016787024594,
-0.0203050770794431));
#44978=CARTESIAN_POINT('Ctrl Pts',(-0.0160934832388148,-0.0421081666096336,
-0.0202337996395943));
#44979=CARTESIAN_POINT('Ctrl Pts',(-0.0161814674256214,-0.041922448903203,
-0.0201366925151593));
#44980=CARTESIAN_POINT('Ctrl Pts',(-0.0162000031195218,-0.0417853494458315,
-0.0200964174636605));
#44981=CARTESIAN_POINT('Ctrl Pts',(-0.0161999999992124,-0.0417115113138095,
-0.0200722578454137));
#44982=CARTESIAN_POINT('Ctrl Pts',(-0.0159803330326857,-0.042259107422558,
-0.0200214959165956));
#44983=CARTESIAN_POINT('Ctrl Pts',(-0.0160240415983998,-0.0422153978669277,
-0.0200134117755617));
#44984=CARTESIAN_POINT('Ctrl Pts',(-0.0161023983074396,-0.0421153793218915,
-0.0199958012406195));
#44985=CARTESIAN_POINT('Ctrl Pts',(-0.016180854669548,-0.0419335087707168,
-0.019967423336514));
#44986=CARTESIAN_POINT('Ctrl Pts',(-0.0162000032226061,-0.0417978396108662,
-0.0199498751917828));
#44987=CARTESIAN_POINT('Ctrl Pts',(-0.0161999999991864,-0.0417287424088398,
-0.0199413801943158));
#44988=CARTESIAN_POINT('Ctrl Pts',(-0.0159803300851459,-0.0422591044750182,
-0.0198758930429547));
#44989=CARTESIAN_POINT('Ctrl Pts',(-0.0160266114141904,-0.0422128231462237,
-0.0198758971261998));
#44990=CARTESIAN_POINT('Ctrl Pts',(-0.0161069828280334,-0.0421080797083306,
-0.0198759060213743));
#44991=CARTESIAN_POINT('Ctrl Pts',(-0.0161827725636957,-0.041925103292344,
-0.0198759203544499));
#44992=CARTESIAN_POINT('Ctrl Pts',(-0.0162000028998043,-0.0417942003715057,
-0.0198759292168042));
#44993=CARTESIAN_POINT('Ctrl Pts',(-0.0161999999992679,-0.0417287413450437,
-0.0198759335072381));
#44994=CARTESIAN_POINT('',(-0.0159803300858899,-0.0422591044757622,-0.0198759665451098));
#44995=CARTESIAN_POINT('Ctrl Pts',(-0.0157883689863059,-0.0420671433761781,
-0.0209642222728639));
#44996=CARTESIAN_POINT('Ctrl Pts',(-0.0158238948255348,-0.0421026692154071,
-0.020893170594406));
#44997=CARTESIAN_POINT('Ctrl Pts',(-0.0158828523983345,-0.0421616267882068,
-0.020739486498496));
#44998=CARTESIAN_POINT('Ctrl Pts',(-0.0159628190767039,-0.0422415934665763,
-0.0203355262744823));
#44999=CARTESIAN_POINT('Ctrl Pts',(-0.0159803300858999,-0.0422591044757722,
-0.0200215487583781));
#45000=CARTESIAN_POINT('Ctrl Pts',(-0.0159803300858999,-0.0422591044757722,
-0.0198759665451198));
#45001=CARTESIAN_POINT('',(-0.0162,-0.0417287743898723,-0.0198759665451098));
#45002=CARTESIAN_POINT('Origin',(-0.01545000000001,-0.0417287743898823,
-0.0198759665451198));
#45003=CARTESIAN_POINT('Origin',(-0.01620000000001,-0.040978887648414,-0.0198759665451198));
#45004=CARTESIAN_POINT('Ctrl Pts',(-0.0157883510491115,-0.0420671254389838,
-0.0209642581457028));
#45005=CARTESIAN_POINT('Ctrl Pts',(-0.0158238849031055,-0.0421026592929779,
-0.0208931964581408));
#45006=CARTESIAN_POINT('Ctrl Pts',(-0.0158828479122753,-0.0421616223021476,
-0.0207395091602429));
#45007=CARTESIAN_POINT('Ctrl Pts',(-0.0159628235627431,-0.0422415979526155,
-0.0203355036127154));
#45008=CARTESIAN_POINT('Ctrl Pts',(-0.0159803330326857,-0.042259107422558,
-0.0200214959165957));
#45009=CARTESIAN_POINT('Ctrl Pts',(-0.0159803300851459,-0.0422591044750182,
-0.0198758930429548));
#45010=CARTESIAN_POINT('Ctrl Pts',(-0.0157528254319759,-0.0421381807912529,
-0.0209287319941251));
#45011=CARTESIAN_POINT('Ctrl Pts',(-0.0157879192374369,-0.0421664366105106,
-0.0208582891550461));
#45012=CARTESIAN_POINT('Ctrl Pts',(-0.0158470801331242,-0.0422151679902413,
-0.0207046736936446));
#45013=CARTESIAN_POINT('Ctrl Pts',(-0.0159229043125871,-0.0422873985837833,
-0.0203050770794431));
#45014=CARTESIAN_POINT('Ctrl Pts',(-0.0159366234770554,-0.0423028159882721,
-0.0200134117755617));
#45015=CARTESIAN_POINT('Ctrl Pts',(-0.0159340487563514,-0.0423053858040627,
-0.0198758971261998));
#45016=CARTESIAN_POINT('Ctrl Pts',(-0.0156743980241005,-0.0422592722231821,
-0.0208503044065784));
#45017=CARTESIAN_POINT('Ctrl Pts',(-0.0157091531723958,-0.0422778860192916,
-0.0207798791280559));
#45018=CARTESIAN_POINT('Ctrl Pts',(-0.0157672464104802,-0.0423135447464294,
-0.0206223860725731));
#45019=CARTESIAN_POINT('Ctrl Pts',(-0.0158293922197613,-0.042372257628687,
-0.0202337996395943));
#45020=CARTESIAN_POINT('Ctrl Pts',(-0.0158366049320192,-0.0423811726973118,
-0.0199958012406195));
#45021=CARTESIAN_POINT('Ctrl Pts',(-0.0158293053184583,-0.0423857572179058,
-0.0198759060213744));
#45022=CARTESIAN_POINT('Ctrl Pts',(-0.015468305878648,-0.042427406620866,
-0.0206442137889348));
#45023=CARTESIAN_POINT('Ctrl Pts',(-0.0155066139651701,-0.0424344514374237,
-0.0205743150054965));
#45024=CARTESIAN_POINT('Ctrl Pts',(-0.0155701075544921,-0.0424501760183725,
-0.0204151632671822));
#45025=CARTESIAN_POINT('Ctrl Pts',(-0.0156436745133307,-0.0424602418154937,
-0.0201366925151594));
#45026=CARTESIAN_POINT('Ctrl Pts',(-0.0156547343808444,-0.0424596290594203,
-0.019967423336514));
#45027=CARTESIAN_POINT('Ctrl Pts',(-0.0156463289024716,-0.042461546953568,
-0.0198759203544499));
#45028=CARTESIAN_POINT('Ctrl Pts',(-0.0153031099239469,-0.0424787830360672,
-0.0204790137545434));
#45029=CARTESIAN_POINT('Ctrl Pts',(-0.0153491317045512,-0.0424787818503417,
-0.0204249098239339));
#45030=CARTESIAN_POINT('Ctrl Pts',(-0.015429515552737,-0.0424787792037377,
-0.0203052594890441));
#45031=CARTESIAN_POINT('Ctrl Pts',(-0.0155065750559592,-0.0424787775093941,
-0.0200964174636605));
#45032=CARTESIAN_POINT('Ctrl Pts',(-0.0155190652209939,-0.0424787776124784,
-0.0199498751917829));
#45033=CARTESIAN_POINT('Ctrl Pts',(-0.0155154259816334,-0.0424787772896766,
-0.0198759292168042));
#45034=CARTESIAN_POINT('Ctrl Pts',(-0.0152303031410804,-0.0424787743876895,
-0.0204062031513794));
#45035=CARTESIAN_POINT('Ctrl Pts',(-0.0152765861541423,-0.0424787743879888,
-0.0203599283242667));
#45036=CARTESIAN_POINT('Ctrl Pts',(-0.0153569536803697,-0.042478774388657,
-0.0202552032610877));
#45037=CARTESIAN_POINT('Ctrl Pts',(-0.0154327369239373,-0.0424787743890847,
-0.0200722578454137));
#45038=CARTESIAN_POINT('Ctrl Pts',(-0.0154499680189675,-0.0424787743890587,
-0.0199413801943158));
#45039=CARTESIAN_POINT('Ctrl Pts',(-0.0154499669551714,-0.0424787743891402,
-0.0198759335072381));
#45040=CARTESIAN_POINT('',(-0.0152303632585517,-0.0424787743898723,-0.0204062165451098));
#45041=CARTESIAN_POINT('Ctrl Pts',(-0.0157883689863059,-0.0420671433761781,
-0.0209642222728639));
#45042=CARTESIAN_POINT('Ctrl Pts',(-0.0157528431470768,-0.0421381950546361,
-0.020928696433635));
#45043=CARTESIAN_POINT('Ctrl Pts',(-0.0156744155682287,-0.0422592816194792,
-0.0208502688547868));
#45044=CARTESIAN_POINT('Ctrl Pts',(-0.0154683367770566,-0.0424274007458997,
-0.0206441900636147));
#45045=CARTESIAN_POINT('Ctrl Pts',(-0.0153031609543063,-0.0424787743898823,
-0.0204790142408644));
#45046=CARTESIAN_POINT('Ctrl Pts',(-0.0152303632585616,-0.0424787743898823,
-0.0204062165451198));
#45047=CARTESIAN_POINT('',(-0.01545,-0.0424787743898723,-0.0198759665451098));
#45048=CARTESIAN_POINT('Origin',(-0.0147001132585417,-0.0424787743898823,
-0.0198759665451198));
#45049=CARTESIAN_POINT('Origin',(-0.01545000000001,-0.0417287743898823,
-0.0198759665451198));
#45050=CARTESIAN_POINT('Ctrl Pts',(-0.0157884048591437,-0.0420671254389844,
-0.0209642043356702));
#45051=CARTESIAN_POINT('Ctrl Pts',(-0.0157528787075659,-0.0421381807912533,
-0.0209286787185346));
#45052=CARTESIAN_POINT('Ctrl Pts',(-0.0156744511200192,-0.0422592722231824,
-0.0208502513106591));
#45053=CARTESIAN_POINT('Ctrl Pts',(-0.0154683605023777,-0.0424274066208644,
-0.0206441591652087));
#45054=CARTESIAN_POINT('Ctrl Pts',(-0.0153031604679893,-0.0424787830360656,
-0.0204789632105105));
#45055=CARTESIAN_POINT('Ctrl Pts',(-0.015230349864827,-0.0424787743876894,
-0.0204061564276457));
#45056=CARTESIAN_POINT('Ctrl Pts',(-0.0157173431715819,-0.0421026592929782,
-0.0209997381896639));
#45057=CARTESIAN_POINT('Ctrl Pts',(-0.0156824358684873,-0.0421664366105109,
-0.0209637725239953));
#45058=CARTESIAN_POINT('Ctrl Pts',(-0.015604025841497,-0.0422778860192918,
-0.0208850064589542));
#45059=CARTESIAN_POINT('Ctrl Pts',(-0.0153984617189395,-0.0424344514374223,
-0.0206824672517305));
#45060=CARTESIAN_POINT('Ctrl Pts',(-0.0152490565373796,-0.0424787818503404,
-0.0205249849911143));
#45061=CARTESIAN_POINT('Ctrl Pts',(-0.0151840750377138,-0.0424787743879888,
-0.0204524394407073));
#45062=CARTESIAN_POINT('Ctrl Pts',(-0.0155636558736842,-0.0421616223021478,
-0.0210587011988336));
#45063=CARTESIAN_POINT('Ctrl Pts',(-0.0155288204070858,-0.0422151679902414,
-0.0210229334196824));
#45064=CARTESIAN_POINT('Ctrl Pts',(-0.0154465327860143,-0.0423135447464295,
-0.0209430996970383));
#45065=CARTESIAN_POINT('Ctrl Pts',(-0.0152393099806257,-0.0424501760183712,
-0.0207459608410522));
#45066=CARTESIAN_POINT('Ctrl Pts',(-0.0151294062024889,-0.0424787792037368,
-0.0206053688392994));
#45067=CARTESIAN_POINT('Ctrl Pts',(-0.0150793499745336,-0.042478774388657,
-0.0205328069669344));
#45068=CARTESIAN_POINT('Ctrl Pts',(-0.0151596503261579,-0.0422415979526153,
-0.0211386768493011));
#45069=CARTESIAN_POINT('Ctrl Pts',(-0.0151292237928857,-0.0422873985837832,
-0.0210987575991451));
#45070=CARTESIAN_POINT('Ctrl Pts',(-0.0150579463530369,-0.0423722576286868,
-0.0210052455063194));
#45071=CARTESIAN_POINT('Ctrl Pts',(-0.0149608392286026,-0.0424602418154928,
-0.0208195277998905));
#45072=CARTESIAN_POINT('Ctrl Pts',(-0.0149205641771039,-0.0424787775093935,
-0.0206824283425213));
#45073=CARTESIAN_POINT('Ctrl Pts',(-0.014896404558858,-0.0424787743890847,
-0.0206085902105018));
#45074=CARTESIAN_POINT('Ctrl Pts',(-0.0148456426300391,-0.0422591074225579,
-0.0211561863192437));
#45075=CARTESIAN_POINT('Ctrl Pts',(-0.0148375584890051,-0.042302815988272,
-0.0211124767636134));
#45076=CARTESIAN_POINT('Ctrl Pts',(-0.0148199479540626,-0.0423811726973118,
-0.0210124582185773));
#45077=CARTESIAN_POINT('Ctrl Pts',(-0.0147915700499571,-0.0424596290594196,
-0.0208305876674042));
#45078=CARTESIAN_POINT('Ctrl Pts',(-0.014774021905226,-0.0424787776124778,
-0.0206949185075559));
#45079=CARTESIAN_POINT('Ctrl Pts',(-0.0147655269077591,-0.0424787743890587,
-0.0206258213055317));
#45080=CARTESIAN_POINT('Ctrl Pts',(-0.0147000397563989,-0.0422591044750182,
-0.021156183371704));
#45081=CARTESIAN_POINT('Ctrl Pts',(-0.0147000438396438,-0.0423053858040627,
-0.0211099020429095));
#45082=CARTESIAN_POINT('Ctrl Pts',(-0.0147000527348181,-0.0423857572179057,
-0.0210051586050165));
#45083=CARTESIAN_POINT('Ctrl Pts',(-0.0147000670678932,-0.0424615469535673,
-0.0208221821890316));
#45084=CARTESIAN_POINT('Ctrl Pts',(-0.0147000759302473,-0.0424787772896761,
-0.0206912792681954));
#45085=CARTESIAN_POINT('Ctrl Pts',(-0.014700080220681,-0.0424787743891402,
-0.0206258202417353));
#45086=CARTESIAN_POINT('',(-0.0147001132585517,-0.0422591044757622,-0.021156183372448));
#45087=CARTESIAN_POINT('Ctrl Pts',(-0.0157883689863059,-0.0420671433761781,
-0.0209642222728639));
#45088=CARTESIAN_POINT('Ctrl Pts',(-0.0157173173078478,-0.0421026692154071,
-0.0209997481120929));
#45089=CARTESIAN_POINT('Ctrl Pts',(-0.0155636332119379,-0.0421616267882068,
-0.0210587056848926));
#45090=CARTESIAN_POINT('Ctrl Pts',(-0.0151596729879242,-0.0422415934665763,
-0.0211386723632621));
#45091=CARTESIAN_POINT('Ctrl Pts',(-0.0148456954718,-0.0422591044757722,
-0.021156183372458));
#45092=CARTESIAN_POINT('Ctrl Pts',(-0.0147001132585417,-0.0422591044757722,
-0.021156183372458));
#45093=CARTESIAN_POINT('',(-0.0147001132585517,-0.0424787743898723,-0.0206258532865581));
#45094=CARTESIAN_POINT('Origin',(-0.0147001132585417,-0.0417287743898823,
-0.0206258532865681));
#45095=CARTESIAN_POINT('Origin',(-0.0147001132585417,-0.0424787743898823,
-0.0198759665451198));
#45096=CARTESIAN_POINT('Ctrl Pts',(-0.0157884048591435,-0.0420671254389844,
-0.0209642043356702));
#45097=CARTESIAN_POINT('Ctrl Pts',(-0.0157173431715818,-0.0421026592929782,
-0.020999738189664));
#45098=CARTESIAN_POINT('Ctrl Pts',(-0.0155636558736841,-0.0421616223021478,
-0.0210587011988336));
#45099=CARTESIAN_POINT('Ctrl Pts',(-0.015159650326158,-0.0422415979526153,
-0.0211386768493011));
#45100=CARTESIAN_POINT('Ctrl Pts',(-0.0148456426300393,-0.0422591074225579,
-0.0211561863192437));
#45101=CARTESIAN_POINT('Ctrl Pts',(-0.0147000397563992,-0.0422591044750182,
-0.021156183371704));
#45102=CARTESIAN_POINT('Ctrl Pts',(-0.0157528787075658,-0.0420315998218488,
-0.0210352596879392));
#45103=CARTESIAN_POINT('Ctrl Pts',(-0.0156824358684872,-0.0420666936273096,
-0.0210635155071967));
#45104=CARTESIAN_POINT('Ctrl Pts',(-0.0155288204070858,-0.0421258545229966,
-0.0211122468869272));
#45105=CARTESIAN_POINT('Ctrl Pts',(-0.0151292237928857,-0.0422016787024593,
-0.021184477480469));
#45106=CARTESIAN_POINT('Ctrl Pts',(-0.0148375584890053,-0.0422153978669276,
-0.0211998948849578));
#45107=CARTESIAN_POINT('Ctrl Pts',(-0.0147000438396441,-0.0422128231462237,
-0.0212024647007484));
#45108=CARTESIAN_POINT('Ctrl Pts',(-0.0156744511200191,-0.0419531724139732,
-0.0211563511198682));
#45109=CARTESIAN_POINT('Ctrl Pts',(-0.0156040258414969,-0.0419879275622684,
-0.0211749649159776));
#45110=CARTESIAN_POINT('Ctrl Pts',(-0.0154465327860142,-0.0420460208003526,
-0.0212106236431153));
#45111=CARTESIAN_POINT('Ctrl Pts',(-0.015057946353037,-0.0421081666096335,
-0.0212693365253727));
#45112=CARTESIAN_POINT('Ctrl Pts',(-0.0148199479540628,-0.0421153793218915,
-0.0212782515939976));
#45113=CARTESIAN_POINT('Ctrl Pts',(-0.0147000527348183,-0.0421080797083307,
-0.0212828361145914));
#45114=CARTESIAN_POINT('Ctrl Pts',(-0.0154683605023745,-0.0417470802685199,
-0.0213244855175527));
#45115=CARTESIAN_POINT('Ctrl Pts',(-0.0153984617189363,-0.0417853883550417,
-0.0213315303341105));
#45116=CARTESIAN_POINT('Ctrl Pts',(-0.0152393099806225,-0.0418488819443635,
-0.021347254915059));
#45117=CARTESIAN_POINT('Ctrl Pts',(-0.0149608392286012,-0.0419224489032019,
-0.0213573207121799));
#45118=CARTESIAN_POINT('Ctrl Pts',(-0.0147915700499568,-0.0419335087707158,
-0.0213567079561065));
#45119=CARTESIAN_POINT('Ctrl Pts',(-0.0147000670678934,-0.0419251032923431,
-0.0213586258502542));
#45120=CARTESIAN_POINT('Ctrl Pts',(-0.0153031604679818,-0.0415818843138173,
-0.0213758619327538));
#45121=CARTESIAN_POINT('Ctrl Pts',(-0.0152490565373728,-0.0416279060944215,
-0.0213758607470282));
#45122=CARTESIAN_POINT('Ctrl Pts',(-0.0151294062024839,-0.0417082899426073,
-0.021375858100424));
#45123=CARTESIAN_POINT('Ctrl Pts',(-0.0149205641771022,-0.0417853494458292,
-0.0213758564060802));
#45124=CARTESIAN_POINT('Ctrl Pts',(-0.0147740219052253,-0.041797839610864,
-0.0213758565091645));
#45125=CARTESIAN_POINT('Ctrl Pts',(-0.0147000759302474,-0.0417942003715037,
-0.0213758561863626));
#45126=CARTESIAN_POINT('Ctrl Pts',(-0.0152303498648171,-0.0415090775309501,
-0.0213758532843752));
#45127=CARTESIAN_POINT('Ctrl Pts',(-0.0151840750377049,-0.0415553605440118,
-0.0213758532846746));
#45128=CARTESIAN_POINT('Ctrl Pts',(-0.0150793499745268,-0.0416357280702388,
-0.0213758532853428));
#45129=CARTESIAN_POINT('Ctrl Pts',(-0.0148964045588548,-0.041711511313806,
-0.0213758532857705));
#45130=CARTESIAN_POINT('Ctrl Pts',(-0.014765526907758,-0.0417287424088365,
-0.0213758532857445));
#45131=CARTESIAN_POINT('Ctrl Pts',(-0.0147000802206811,-0.0417287413450406,
-0.021375853285826));
#45132=CARTESIAN_POINT('',(-0.0152303632585517,-0.041509137648424,-0.0213758532865581));
#45133=CARTESIAN_POINT('Ctrl Pts',(-0.0157883689863059,-0.0420671433761781,
-0.0209642222728639));
#45134=CARTESIAN_POINT('Ctrl Pts',(-0.0157528431470768,-0.0420316175369492,
-0.0210352739513219));
#45135=CARTESIAN_POINT('Ctrl Pts',(-0.0156744155682287,-0.0419531899581009,
-0.021156360516165));
#45136=CARTESIAN_POINT('Ctrl Pts',(-0.0154683367770566,-0.0417471111669288,
-0.0213244796425855));
#45137=CARTESIAN_POINT('Ctrl Pts',(-0.0153031609543063,-0.0415819353441785,
-0.0213758532865681));
#45138=CARTESIAN_POINT('Ctrl Pts',(-0.0152303632585616,-0.041509137648434,
-0.0213758532865681));
#45139=CARTESIAN_POINT('',(-0.0147001132585517,-0.0417287743898723,-0.0213758532865581));
#45140=CARTESIAN_POINT('Origin',(-0.0147001132585417,-0.040978887648414,
-0.0213758532865681));
#45141=CARTESIAN_POINT('Origin',(-0.0147001132585417,-0.0417287743898823,
-0.0206258532865681));
#45142=CARTESIAN_POINT('Ctrl Pts',(0.00878835104911206,-0.042067179249016,
-0.0209642043356701));
#45143=CARTESIAN_POINT('Ctrl Pts',(0.00882388490310584,-0.0419961175614543,
-0.0209997381896639));
#45144=CARTESIAN_POINT('Ctrl Pts',(0.00888284791227546,-0.0418424302635564,
-0.0210587011988336));
#45145=CARTESIAN_POINT('Ctrl Pts',(0.00896282356274304,-0.0414384247160302,
-0.0211386768493011));
#45146=CARTESIAN_POINT('Ctrl Pts',(0.00898033303268563,-0.0411244170199114,
-0.0211561863192437));
#45147=CARTESIAN_POINT('Ctrl Pts',(0.00898033008514593,-0.0409788141462712,
-0.021156183371704));
#45148=CARTESIAN_POINT('Ctrl Pts',(0.00875282543197645,-0.0420316530974382,
-0.0210352596879391));
#45149=CARTESIAN_POINT('Ctrl Pts',(0.00878791923743724,-0.0419612102583595,
-0.0210635155071967));
#45150=CARTESIAN_POINT('Ctrl Pts',(0.00884708013312432,-0.0418075947969582,
-0.0211122468869272));
#45151=CARTESIAN_POINT('Ctrl Pts',(0.00892290431258698,-0.0414079981827579,
-0.021184477480469));
#45152=CARTESIAN_POINT('Ctrl Pts',(0.00893662347705534,-0.0411163328788773,
-0.0211998948849578));
#45153=CARTESIAN_POINT('Ctrl Pts',(0.00893404875635143,-0.0409788182295161,
-0.0212024647007484));
#45154=CARTESIAN_POINT('Ctrl Pts',(0.00867439802410097,-0.0419532255098914,
-0.0211563511198682));
#45155=CARTESIAN_POINT('Ctrl Pts',(0.00870915317239613,-0.0418828002313693,
-0.0211749649159776));
#45156=CARTESIAN_POINT('Ctrl Pts',(0.00876724641048034,-0.0417253071758866,
-0.0212106236431153));
#45157=CARTESIAN_POINT('Ctrl Pts',(0.00882939221976116,-0.0413367207429092,
-0.0212693365253728));
#45158=CARTESIAN_POINT('Ctrl Pts',(0.0088366049320192,-0.0410987223439349,
-0.0212782515939976));
#45159=CARTESIAN_POINT('Ctrl Pts',(0.00882930531845842,-0.0409788271246903,
-0.0212828361145914));
#45160=CARTESIAN_POINT('Ctrl Pts',(0.00846830587865044,-0.04174713489225,
-0.0213244855175502));
#45161=CARTESIAN_POINT('Ctrl Pts',(0.00850661396517239,-0.0416772361088118,
-0.0213315303341082));
#45162=CARTESIAN_POINT('Ctrl Pts',(0.0085701075544941,-0.041518084370498,
-0.021347254915057));
#45163=CARTESIAN_POINT('Ctrl Pts',(0.00864367451333237,-0.0412396136184749,
-0.0213573207121786));
#45164=CARTESIAN_POINT('Ctrl Pts',(0.00865473438084613,-0.0410703444398294,
-0.0213567079561054));
#45165=CARTESIAN_POINT('Ctrl Pts',(0.00864632890247354,-0.0409788414577655,
-0.0213586258502531));
#45166=CARTESIAN_POINT('Ctrl Pts',(0.0083031099239524,-0.0415819348578615,
-0.0213758619327514));
#45167=CARTESIAN_POINT('Ctrl Pts',(0.00834913170455623,-0.0415278309272518,
-0.0213758607470262));
#45168=CARTESIAN_POINT('Ctrl Pts',(0.00842951555274124,-0.0414081805923612,
-0.0213758581004227));
#45169=CARTESIAN_POINT('Ctrl Pts',(0.00850657505596321,-0.0411993385669761,
-0.0213758564060794));
#45170=CARTESIAN_POINT('Ctrl Pts',(0.0085190652209978,-0.0410527962950982,
-0.0213758565091637));
#45171=CARTESIAN_POINT('Ctrl Pts',(0.00851542598163732,-0.0409788503201196,
-0.0213758561863619));
#45172=CARTESIAN_POINT('Ctrl Pts',(0.00823030314108753,-0.0415091242546993,
-0.0213758532843753));
#45173=CARTESIAN_POINT('Ctrl Pts',(0.00827658615414917,-0.0414628494275861,
-0.0213758532846746));
#45174=CARTESIAN_POINT('Ctrl Pts',(0.00835695368037628,-0.041358124364406,
-0.0213758532853428));
#45175=CARTESIAN_POINT('Ctrl Pts',(0.00843273692394364,-0.0411751789487302,
-0.0213758532857705));
#45176=CARTESIAN_POINT('Ctrl Pts',(0.00844996801897354,-0.0410443012976313,
-0.0213758532857445));
#45177=CARTESIAN_POINT('Ctrl Pts',(0.0084499669551772,-0.0409788546105533,
-0.021375853285826));
#45178=CARTESIAN_POINT('',(0.0087883689862958,-0.0420671433761681,-0.0209642222728539));
#45179=CARTESIAN_POINT('',(0.0089803300858899,-0.040978887648424,-0.021156183372448));
#45180=CARTESIAN_POINT('Ctrl Pts',(0.0087883689863058,-0.0420671433761781,
-0.0209642222728639));
#45181=CARTESIAN_POINT('Ctrl Pts',(0.0088238948255348,-0.0419960916977202,
-0.0209997481120929));
#45182=CARTESIAN_POINT('Ctrl Pts',(0.0088828523983345,-0.0418424076018101,
-0.0210587056848926));
#45183=CARTESIAN_POINT('Ctrl Pts',(0.008962819076704,-0.0414384473777965,
-0.0211386723632621));
#45184=CARTESIAN_POINT('Ctrl Pts',(0.0089803300858999,-0.0411244698616723,
-0.021156183372458));
#45185=CARTESIAN_POINT('Ctrl Pts',(0.0089803300858999,-0.040978887648414,
-0.021156183372458));
#45186=CARTESIAN_POINT('',(0.0082303632585517,-0.041509137648424,-0.0213758532865581));
#45187=CARTESIAN_POINT('Ctrl Pts',(0.0087883689863058,-0.0420671433761781,
-0.0209642222728639));
#45188=CARTESIAN_POINT('Ctrl Pts',(0.0087528431470769,-0.0420316175369492,
-0.0210352739513219));
#45189=CARTESIAN_POINT('Ctrl Pts',(0.0086744155682287,-0.0419531899581009,
-0.021156360516165));
#45190=CARTESIAN_POINT('Ctrl Pts',(0.0084683367770565,-0.0417471111669288,
-0.0213244796425855));
#45191=CARTESIAN_POINT('Ctrl Pts',(0.0083031609543063,-0.0415819353441785,
-0.0213758532865681));
#45192=CARTESIAN_POINT('Ctrl Pts',(0.0082303632585617,-0.041509137648434,
-0.0213758532865681));
#45193=CARTESIAN_POINT('',(0.00845,-0.040978887648424,-0.0213758532865581));
#45194=CARTESIAN_POINT('Origin',(0.0077001132585617,-0.040978887648414,
-0.0213758532865681));
#45195=CARTESIAN_POINT('Origin',(0.00845000000001,-0.040978887648414,-0.0206258532865681));
#45196=CARTESIAN_POINT('Ctrl Pts',(0.00878840485914476,-0.0420671254389838,
-0.0209642043356696));
#45197=CARTESIAN_POINT('Ctrl Pts',(0.00875287870756702,-0.0420315998218482,
-0.0210352596879387));
#45198=CARTESIAN_POINT('Ctrl Pts',(0.00867445112002032,-0.0419531724139726,
-0.0211563511198679));
#45199=CARTESIAN_POINT('Ctrl Pts',(0.00846836050237665,-0.0417470802685202,
-0.0213244855175518));
#45200=CARTESIAN_POINT('Ctrl Pts',(0.00830316046798527,-0.041581884313819,
-0.021375861932753));
#45201=CARTESIAN_POINT('Ctrl Pts',(0.00823034986482127,-0.0415090775309527,
-0.0213758532843752));
#45202=CARTESIAN_POINT('Ctrl Pts',(0.00871734317158273,-0.0421026592929779,
-0.0209997381896636));
#45203=CARTESIAN_POINT('Ctrl Pts',(0.00868243586848799,-0.0420666936273092,
-0.0210635155071964));
#45204=CARTESIAN_POINT('Ctrl Pts',(0.00860402584149779,-0.041987927562268,
-0.0211749649159774));
#45205=CARTESIAN_POINT('Ctrl Pts',(0.0083984617189383,-0.0417853883550424,
-0.0213315303341096));
#45206=CARTESIAN_POINT('Ctrl Pts',(0.00824905653737567,-0.0416279060944235,
-0.0213758607470275));
#45207=CARTESIAN_POINT('Ctrl Pts',(0.00818407503770855,-0.0415553605440146,
-0.0213758532846746));
#45208=CARTESIAN_POINT('Ctrl Pts',(0.00856365587368485,-0.0421616223021476,
-0.0210587011988334));
#45209=CARTESIAN_POINT('Ctrl Pts',(0.00852882040708653,-0.0421258545229965,
-0.0211122468869271));
#45210=CARTESIAN_POINT('Ctrl Pts',(0.00844653278601498,-0.0420460208003524,
-0.0212106236431152));
#45211=CARTESIAN_POINT('Ctrl Pts',(0.00823930998062413,-0.0418488819443643,
-0.0213472549150583));
#45212=CARTESIAN_POINT('Ctrl Pts',(0.008129406202486,-0.0417082899426094,
-0.0213758581004235));
#45213=CARTESIAN_POINT('Ctrl Pts',(0.0080793499745296,-0.041635728070242,
-0.0213758532853428));
#45214=CARTESIAN_POINT('Ctrl Pts',(0.00815965032615725,-0.0422415979526155,
-0.0211386768493013));
#45215=CARTESIAN_POINT('Ctrl Pts',(0.00812922379288497,-0.0422016787024594,
-0.0211844774804691));
#45216=CARTESIAN_POINT('Ctrl Pts',(0.00805794635303622,-0.0421081666096336,
-0.0212693365253729));
#45217=CARTESIAN_POINT('Ctrl Pts',(0.00796083922860117,-0.041922448903203,
-0.0213573207121794));
#45218=CARTESIAN_POINT('Ctrl Pts',(0.00792056417710239,-0.0417853494458315,
-0.0213758564060799));
#45219=CARTESIAN_POINT('Ctrl Pts',(0.00789640455885557,-0.0417115113138095,
-0.0213758532857705));
#45220=CARTESIAN_POINT('Ctrl Pts',(0.00784564263003751,-0.042259107422558,
-0.0211561863192438));
#45221=CARTESIAN_POINT('Ctrl Pts',(0.00783755848900357,-0.0422153978669277,
-0.0211998948849579));
#45222=CARTESIAN_POINT('Ctrl Pts',(0.00781994795406137,-0.0421153793218915,
-0.0212782515939977));
#45223=CARTESIAN_POINT('Ctrl Pts',(0.00779157004995592,-0.0419335087707168,
-0.0213567079561061));
#45224=CARTESIAN_POINT('Ctrl Pts',(0.00777402190522474,-0.0417978396108662,
-0.0213758565091642));
#45225=CARTESIAN_POINT('Ctrl Pts',(0.00776552690775767,-0.0417287424088398,
-0.0213758532857445));
#45226=CARTESIAN_POINT('Ctrl Pts',(0.00770003975639664,-0.0422591044750182,
-0.021156183371704));
#45227=CARTESIAN_POINT('Ctrl Pts',(0.00770004383964167,-0.0422128231462237,
-0.0212024647007485));
#45228=CARTESIAN_POINT('Ctrl Pts',(0.00770005273481621,-0.0421080797083306,
-0.0212828361145915));
#45229=CARTESIAN_POINT('Ctrl Pts',(0.0077000670678918,-0.0419251032923439,
-0.0213586258502538));
#45230=CARTESIAN_POINT('Ctrl Pts',(0.00770007593024611,-0.0417942003715057,
-0.0213758561863624));
#45231=CARTESIAN_POINT('Ctrl Pts',(0.00770008022067996,-0.0417287413450437,
-0.021375853285826));
#45232=CARTESIAN_POINT('',(0.0077001132585517,-0.0422591044757622,-0.021156183372448));
#45233=CARTESIAN_POINT('Ctrl Pts',(0.0087883689863058,-0.0420671433761781,
-0.0209642222728639));
#45234=CARTESIAN_POINT('Ctrl Pts',(0.0087173173078479,-0.0421026692154071,
-0.0209997481120929));
#45235=CARTESIAN_POINT('Ctrl Pts',(0.0085636332119379,-0.0421616267882068,
-0.0210587056848926));
#45236=CARTESIAN_POINT('Ctrl Pts',(0.0081596729879242,-0.0422415934665763,
-0.0211386723632621));
#45237=CARTESIAN_POINT('Ctrl Pts',(0.00784569547182,-0.0422591044757722,
-0.021156183372458));
#45238=CARTESIAN_POINT('Ctrl Pts',(0.0077001132585617,-0.0422591044757722,
-0.021156183372458));
#45239=CARTESIAN_POINT('',(0.0077001132585517,-0.0417287743898723,-0.0213758532865581));
#45240=CARTESIAN_POINT('Origin',(0.0077001132585617,-0.0417287743898823,
-0.0206258532865681));
#45241=CARTESIAN_POINT('Origin',(0.0077001132585617,-0.040978887648414,
-0.0213758532865681));
#45242=CARTESIAN_POINT('Ctrl Pts',(0.00878840485914491,-0.0420671254389837,
-0.0209642043356696));
#45243=CARTESIAN_POINT('Ctrl Pts',(0.00871734317158283,-0.0421026592929778,
-0.0209997381896636));
#45244=CARTESIAN_POINT('Ctrl Pts',(0.00856365587368494,-0.0421616223021476,
-0.0210587011988334));
#45245=CARTESIAN_POINT('Ctrl Pts',(0.00815965032615716,-0.0422415979526155,
-0.0211386768493013));
#45246=CARTESIAN_POINT('Ctrl Pts',(0.0078456426300373,-0.042259107422558,
-0.0211561863192438));
#45247=CARTESIAN_POINT('Ctrl Pts',(0.00770003975639635,-0.0422591044750182,
-0.021156183371704));
#45248=CARTESIAN_POINT('Ctrl Pts',(0.00875287870756717,-0.0421381807912528,
-0.0209286787185338));
#45249=CARTESIAN_POINT('Ctrl Pts',(0.00868243586848809,-0.0421664366105106,
-0.020963772523995));
#45250=CARTESIAN_POINT('Ctrl Pts',(0.00852882040708662,-0.0422151679902413,
-0.0210229334196823));
#45251=CARTESIAN_POINT('Ctrl Pts',(0.00812922379288488,-0.0422873985837833,
-0.0210987575991452));
#45252=CARTESIAN_POINT('Ctrl Pts',(0.00783755848900338,-0.0423028159882721,
-0.0211124767636135));
#45253=CARTESIAN_POINT('Ctrl Pts',(0.00770004383964139,-0.0423053858040627,
-0.0211099020429095));
#45254=CARTESIAN_POINT('Ctrl Pts',(0.00867445112002046,-0.0422592722231821,
-0.0208502513106585));
#45255=CARTESIAN_POINT('Ctrl Pts',(0.00860402584149789,-0.0422778860192916,
-0.0208850064589539));
#45256=CARTESIAN_POINT('Ctrl Pts',(0.00844653278601506,-0.0423135447464294,
-0.0209430996970382));
#45257=CARTESIAN_POINT('Ctrl Pts',(0.00805794635303614,-0.042372257628687,
-0.0210052455063195));
#45258=CARTESIAN_POINT('Ctrl Pts',(0.00781994795406121,-0.0423811726973118,
-0.0210124582185773));
#45259=CARTESIAN_POINT('Ctrl Pts',(0.00770005273481597,-0.0423857572179058,
-0.0210051586050164));
#45260=CARTESIAN_POINT('Ctrl Pts',(0.00846836050238168,-0.042427406620862,
-0.0206441591652107));
#45261=CARTESIAN_POINT('Ctrl Pts',(0.00839846171894318,-0.0424344514374201,
-0.0206824672517328));
#45262=CARTESIAN_POINT('Ctrl Pts',(0.008239309980629,-0.0424501760183693,
-0.0207459608410547));
#45263=CARTESIAN_POINT('Ctrl Pts',(0.00796083922860346,-0.0424602418154917,
-0.0208195277998931));
#45264=CARTESIAN_POINT('Ctrl Pts',(0.00779157004995647,-0.0424596290594185,
-0.0208305876674068));
#45265=CARTESIAN_POINT('Ctrl Pts',(0.00770006706789161,-0.0424615469535663,
-0.0208221821890339));
#45266=CARTESIAN_POINT('Ctrl Pts',(0.00830316046799688,-0.0424787830360636,
-0.0204789632105163));
#45267=CARTESIAN_POINT('Ctrl Pts',(0.00824905653738625,-0.0424787818503386,
-0.0205249849911202));
#45268=CARTESIAN_POINT('Ctrl Pts',(0.0081294062024937,-0.0424787792037357,
-0.0206053688393048));
#45269=CARTESIAN_POINT('Ctrl Pts',(0.00792056417710514,-0.0424787775093928,
-0.0206824283425269));
#45270=CARTESIAN_POINT('Ctrl Pts',(0.00777402190522587,-0.0424787776124771,
-0.0206949185075614));
#45271=CARTESIAN_POINT('Ctrl Pts',(0.00770007593024596,-0.0424787772896754,
-0.0206912792682006));
#45272=CARTESIAN_POINT('Ctrl Pts',(0.00823034986483657,-0.0424787743876894,
-0.0204061564276536));
#45273=CARTESIAN_POINT('Ctrl Pts',(0.00818407503772218,-0.0424787743879888,
-0.0204524394407155));
#45274=CARTESIAN_POINT('Ctrl Pts',(0.00807934997454009,-0.042478774388657,
-0.0205328069669429));
#45275=CARTESIAN_POINT('Ctrl Pts',(0.00789640455886057,-0.0424787743890847,
-0.0206085902105108));
#45276=CARTESIAN_POINT('Ctrl Pts',(0.00776552690775935,-0.0424787743890587,
-0.02062582130554));
#45277=CARTESIAN_POINT('Ctrl Pts',(0.00770008022067983,-0.0424787743891402,
-0.0206258202417431));
#45278=CARTESIAN_POINT('',(0.0082303632585517,-0.0424787743898723,-0.0204062165451098));
#45279=CARTESIAN_POINT('Ctrl Pts',(0.0087883689863058,-0.0420671433761781,
-0.0209642222728639));
#45280=CARTESIAN_POINT('Ctrl Pts',(0.0087528431470769,-0.0421381950546361,
-0.0209286964336349));
#45281=CARTESIAN_POINT('Ctrl Pts',(0.0086744155682287,-0.0422592816194792,
-0.0208502688547868));
#45282=CARTESIAN_POINT('Ctrl Pts',(0.0084683367770566,-0.0424274007458997,
-0.0206441900636147));
#45283=CARTESIAN_POINT('Ctrl Pts',(0.0083031609543063,-0.0424787743898823,
-0.0204790142408644));
#45284=CARTESIAN_POINT('Ctrl Pts',(0.0082303632585617,-0.0424787743898823,
-0.0204062165451198));
#45285=CARTESIAN_POINT('',(0.0077001132585517,-0.0424787743898723,-0.0206258532865581));
#45286=CARTESIAN_POINT('Origin',(0.0077001132585617,-0.0424787743898823,
-0.0198759665451198));
#45287=CARTESIAN_POINT('Origin',(0.0077001132585617,-0.0417287743898823,
-0.0206258532865681));
#45288=CARTESIAN_POINT('Ctrl Pts',(0.00878835104911144,-0.0420671254389837,
-0.020964258145703));
#45289=CARTESIAN_POINT('Ctrl Pts',(0.00875282543197585,-0.0421381807912528,
-0.0209287319941252));
#45290=CARTESIAN_POINT('Ctrl Pts',(0.00867439802410037,-0.0422592722231821,
-0.0208503044065786));
#45291=CARTESIAN_POINT('Ctrl Pts',(0.00846830587865264,-0.042427406620862,
-0.0206442137889398));
#45292=CARTESIAN_POINT('Ctrl Pts',(0.00830310992395822,-0.0424787830360636,
-0.020479013754555));
#45293=CARTESIAN_POINT('Ctrl Pts',(0.00823030314109548,-0.0424787743876894,
-0.0204062031513947));
#45294=CARTESIAN_POINT('Ctrl Pts',(0.0088238849031055,-0.0421026592929778,
-0.0208931964581409));
#45295=CARTESIAN_POINT('Ctrl Pts',(0.00878791923743691,-0.0421664366105106,
-0.0208582891550462));
#45296=CARTESIAN_POINT('Ctrl Pts',(0.00870915317239579,-0.0422778860192916,
-0.020779879128056));
#45297=CARTESIAN_POINT('Ctrl Pts',(0.00850661396517473,-0.0424344514374201,
-0.0205743150055014));
#45298=CARTESIAN_POINT('Ctrl Pts',(0.00834913170456207,-0.0424787818503386,
-0.0204249098239443));
#45299=CARTESIAN_POINT('Ctrl Pts',(0.00827658615415742,-0.0424787743879888,
-0.0203599283242803));
#45300=CARTESIAN_POINT('Ctrl Pts',(0.00888284791227531,-0.0421616223021476,
-0.020739509160243));
#45301=CARTESIAN_POINT('Ctrl Pts',(0.00884708013312418,-0.0422151679902413,
-0.0207046736936447));
#45302=CARTESIAN_POINT('Ctrl Pts',(0.00876724641048012,-0.0423135447464294,
-0.0206223860725732));
#45303=CARTESIAN_POINT('Ctrl Pts',(0.00857010755449659,-0.0424501760183693,
-0.0204151632671871));
#45304=CARTESIAN_POINT('Ctrl Pts',(0.00842951555274672,-0.0424787792037357,
-0.0203052594890518));
#45305=CARTESIAN_POINT('Ctrl Pts',(0.00835695368038484,-0.042478774388657,
-0.0202552032610982));
#45306=CARTESIAN_POINT('Ctrl Pts',(0.00896282356274319,-0.0422415979526155,
-0.0203355036127153));
#45307=CARTESIAN_POINT('Ctrl Pts',(0.00892290431258713,-0.0422873985837833,
-0.020305077079443));
#45308=CARTESIAN_POINT('Ctrl Pts',(0.00882939221976138,-0.042372257628687,
-0.0202337996395942));
#45309=CARTESIAN_POINT('Ctrl Pts',(0.00864367451333499,-0.0424602418154917,
-0.0201366925151615));
#45310=CARTESIAN_POINT('Ctrl Pts',(0.00850657505596884,-0.0424787775093928,
-0.0200964174636632));
#45311=CARTESIAN_POINT('Ctrl Pts',(0.00843273692395266,-0.0424787743890847,
-0.0200722578454187));
#45312=CARTESIAN_POINT('Ctrl Pts',(0.00898033303268573,-0.042259107422558,
-0.0200214959165954));
#45313=CARTESIAN_POINT('Ctrl Pts',(0.00893662347705542,-0.0423028159882721,
-0.0200134117755615));
#45314=CARTESIAN_POINT('Ctrl Pts',(0.00883660493201924,-0.0423811726973119,
-0.0199958012406193));
#45315=CARTESIAN_POINT('Ctrl Pts',(0.00865473438084872,-0.0424596290594185,
-0.0199674233365146));
#45316=CARTESIAN_POINT('Ctrl Pts',(0.0085190652210033,-0.0424787776124771,
-0.019949875191784));
#45317=CARTESIAN_POINT('Ctrl Pts',(0.00844996801898193,-0.0424787743890587,
-0.0199413801943175));
#45318=CARTESIAN_POINT('Ctrl Pts',(0.00898033008514593,-0.0422591044750182,
-0.0198758930429544));
#45319=CARTESIAN_POINT('Ctrl Pts',(0.00893404875635139,-0.0423053858040627,
-0.0198758971261995));
#45320=CARTESIAN_POINT('Ctrl Pts',(0.0088293053184583,-0.0423857572179058,
-0.0198759060213741));
#45321=CARTESIAN_POINT('Ctrl Pts',(0.00864632890247584,-0.0424615469535663,
-0.0198759203544497));
#45322=CARTESIAN_POINT('Ctrl Pts',(0.0085154259816425,-0.0424787772896754,
-0.0198759292168041));
#45323=CARTESIAN_POINT('Ctrl Pts',(0.00844996695518506,-0.0424787743891402,
-0.0198759335072379));
#45324=CARTESIAN_POINT('',(0.0089803300858899,-0.0422591044757622,-0.0198759665451098));
#45325=CARTESIAN_POINT('Ctrl Pts',(0.0087883689863058,-0.0420671433761781,
-0.0209642222728639));
#45326=CARTESIAN_POINT('Ctrl Pts',(0.0088238948255348,-0.0421026692154071,
-0.020893170594406));
#45327=CARTESIAN_POINT('Ctrl Pts',(0.0088828523983345,-0.0421616267882068,
-0.020739486498496));
#45328=CARTESIAN_POINT('Ctrl Pts',(0.008962819076704,-0.0422415934665763,
-0.0203355262744823));
#45329=CARTESIAN_POINT('Ctrl Pts',(0.0089803300858999,-0.0422591044757722,
-0.0200215487583781));
#45330=CARTESIAN_POINT('Ctrl Pts',(0.0089803300858999,-0.0422591044757722,
-0.0198759665451198));
#45331=CARTESIAN_POINT('',(0.00845,-0.0424787743898723,-0.0198759665451098));
#45332=CARTESIAN_POINT('Origin',(0.00845000000001,-0.0417287743898823,-0.0198759665451198));
#45333=CARTESIAN_POINT('Origin',(0.0077001132585617,-0.0424787743898823,
-0.0198759665451198));
#45334=CARTESIAN_POINT('Ctrl Pts',(0.00878835104911152,-0.0420671254389838,
-0.0209642581457029));
#45335=CARTESIAN_POINT('Ctrl Pts',(0.00882388490310554,-0.0421026592929778,
-0.0208931964581408));
#45336=CARTESIAN_POINT('Ctrl Pts',(0.00888284791227533,-0.0421616223021476,
-0.020739509160243));
#45337=CARTESIAN_POINT('Ctrl Pts',(0.00896282356274317,-0.0422415979526155,
-0.0203355036127153));
#45338=CARTESIAN_POINT('Ctrl Pts',(0.00898033303268572,-0.042259107422558,
-0.0200214959165956));
#45339=CARTESIAN_POINT('Ctrl Pts',(0.00898033008514593,-0.0422591044750182,
-0.0198758930429547));
#45340=CARTESIAN_POINT('Ctrl Pts',(0.00885940640138057,-0.0420315998218482,
-0.020928731994125));
#45341=CARTESIAN_POINT('Ctrl Pts',(0.00888766222063833,-0.0420666936273092,
-0.0208582891550461));
#45342=CARTESIAN_POINT('Ctrl Pts',(0.00893639360036898,-0.0421258545229965,
-0.0207046736936446));
#45343=CARTESIAN_POINT('Ctrl Pts',(0.00900862419391102,-0.0422016787024594,
-0.0203050770794431));
#45344=CARTESIAN_POINT('Ctrl Pts',(0.00902404159839978,-0.0422153978669277,
-0.0200134117755617));
#45345=CARTESIAN_POINT('Ctrl Pts',(0.00902661141419038,-0.0422128231462237,
-0.0198758971261998));
#45346=CARTESIAN_POINT('Ctrl Pts',(0.00898049783330982,-0.0419531724139727,
-0.0208503044065784));
#45347=CARTESIAN_POINT('Ctrl Pts',(0.00899911162941933,-0.041987927562268,
-0.0207798791280559));
#45348=CARTESIAN_POINT('Ctrl Pts',(0.00903477035655714,-0.0420460208003524,
-0.0206223860725731));
#45349=CARTESIAN_POINT('Ctrl Pts',(0.00909348323881476,-0.0421081666096336,
-0.0202337996395943));
#45350=CARTESIAN_POINT('Ctrl Pts',(0.00910239830743954,-0.0421153793218915,
-0.0199958012406195));
#45351=CARTESIAN_POINT('Ctrl Pts',(0.0091069828280335,-0.0421080797083306,
-0.0198759060213743));
#45352=CARTESIAN_POINT('Ctrl Pts',(0.00914863223099365,-0.0417470802685202,
-0.0206442137889348));
#45353=CARTESIAN_POINT('Ctrl Pts',(0.00915567704755152,-0.0417853883550424,
-0.0205743150054964));
#45354=CARTESIAN_POINT('Ctrl Pts',(0.00917140162850022,-0.0418488819443643,
-0.0204151632671822));
#45355=CARTESIAN_POINT('Ctrl Pts',(0.00918146742562141,-0.041922448903203,
-0.0201366925151594));
#45356=CARTESIAN_POINT('Ctrl Pts',(0.00918085466954802,-0.0419335087707168,
-0.019967423336514));
#45357=CARTESIAN_POINT('Ctrl Pts',(0.00918277256369573,-0.0419251032923439,
-0.0198759203544499));
#45358=CARTESIAN_POINT('Ctrl Pts',(0.00920000864619486,-0.041581884313819,
-0.0204790137545434));
#45359=CARTESIAN_POINT('Ctrl Pts',(0.00920000746046942,-0.0416279060944234,
-0.0204249098239339));
#45360=CARTESIAN_POINT('Ctrl Pts',(0.0092000048138654,-0.0417082899426094,
-0.0203052594890441));
#45361=CARTESIAN_POINT('Ctrl Pts',(0.0092000031195218,-0.0417853494458315,
-0.0200964174636605));
#45362=CARTESIAN_POINT('Ctrl Pts',(0.00920000322260612,-0.0417978396108662,
-0.0199498751917828));
#45363=CARTESIAN_POINT('Ctrl Pts',(0.00920000289980427,-0.0417942003715057,
-0.0198759292168042));
#45364=CARTESIAN_POINT('Ctrl Pts',(0.00919999999781715,-0.0415090775309527,
-0.0204062031513794));
#45365=CARTESIAN_POINT('Ctrl Pts',(0.0091999999981165,-0.0415553605440146,
-0.0203599283242666));
#45366=CARTESIAN_POINT('Ctrl Pts',(0.00919999999878466,-0.041635728070242,
-0.0202552032610877));
#45367=CARTESIAN_POINT('Ctrl Pts',(0.00919999999921242,-0.0417115113138095,
-0.0200722578454137));
#45368=CARTESIAN_POINT('Ctrl Pts',(0.0091999999991864,-0.0417287424088398,
-0.0199413801943158));
#45369=CARTESIAN_POINT('Ctrl Pts',(0.00919999999926789,-0.0417287413450437,
-0.0198759335072381));
#45370=CARTESIAN_POINT('',(0.0092,-0.041509137648424,-0.0204062165451098));
#45371=CARTESIAN_POINT('Ctrl Pts',(0.0087883689863058,-0.0420671433761781,
-0.0209642222728639));
#45372=CARTESIAN_POINT('Ctrl Pts',(0.0088594206647638,-0.0420316175369492,
-0.0209286964336349));
#45373=CARTESIAN_POINT('Ctrl Pts',(0.0089805072296069,-0.0419531899581009,
-0.0208502688547868));
#45374=CARTESIAN_POINT('Ctrl Pts',(0.0091486263560274,-0.0417471111669288,
-0.0206441900636146));
#45375=CARTESIAN_POINT('Ctrl Pts',(0.00920000000001,-0.0415819353441785,
-0.0204790142408644));
#45376=CARTESIAN_POINT('Ctrl Pts',(0.00920000000001,-0.041509137648434,
-0.0204062165451198));
#45377=CARTESIAN_POINT('',(0.0092,-0.0417287743898723,-0.0198759665451098));
#45378=CARTESIAN_POINT('Origin',(0.00920000000001,-0.040978887648414,-0.0198759665451198));
#45379=CARTESIAN_POINT('Origin',(0.00845000000001,-0.0417287743898823,-0.0198759665451198));
#45380=CARTESIAN_POINT('Ctrl Pts',(0.00878835104911206,-0.042067179249016,
-0.0209642043356702));
#45381=CARTESIAN_POINT('Ctrl Pts',(0.00885940640138099,-0.0420316530974383,
-0.0209286787185344));
#45382=CARTESIAN_POINT('Ctrl Pts',(0.0089804978333101,-0.0419532255098915,
-0.0208502513106591));
#45383=CARTESIAN_POINT('Ctrl Pts',(0.00914863223099209,-0.04174713489225,
-0.0206441591652086));
#45384=CARTESIAN_POINT('Ctrl Pts',(0.00920000864619334,-0.0415819348578615,
-0.0204789632105105));
#45385=CARTESIAN_POINT('Ctrl Pts',(0.00919999999781715,-0.0415091242546993,
-0.0204061564276456));
#45386=CARTESIAN_POINT('Ctrl Pts',(0.00882388490310584,-0.0419961175614543,
-0.0209997381896639));
#45387=CARTESIAN_POINT('Ctrl Pts',(0.00888766222063857,-0.0419612102583595,
-0.0209637725239953));
#45388=CARTESIAN_POINT('Ctrl Pts',(0.00899911162941951,-0.0418828002313693,
-0.0208850064589542));
#45389=CARTESIAN_POINT('Ctrl Pts',(0.00915567704755005,-0.0416772361088118,
-0.0206824672517305));
#45390=CARTESIAN_POINT('Ctrl Pts',(0.00920000746046811,-0.0415278309272518,
-0.0205249849911143));
#45391=CARTESIAN_POINT('Ctrl Pts',(0.0091999999981165,-0.0414628494275861,
-0.0204524394407073));
#45392=CARTESIAN_POINT('Ctrl Pts',(0.00888284791227546,-0.0418424302635564,
-0.0210587011988336));
#45393=CARTESIAN_POINT('Ctrl Pts',(0.00893639360036911,-0.0418075947969582,
-0.0210229334196824));
#45394=CARTESIAN_POINT('Ctrl Pts',(0.00903477035655724,-0.0417253071758866,
-0.0209430996970383));
#45395=CARTESIAN_POINT('Ctrl Pts',(0.00917140162849889,-0.041518084370498,
-0.0207459608410522));
#45396=CARTESIAN_POINT('Ctrl Pts',(0.00920000481386456,-0.0414081805923612,
-0.0206053688392993));
#45397=CARTESIAN_POINT('Ctrl Pts',(0.00919999999878466,-0.041358124364406,
-0.0205328069669344));
#45398=CARTESIAN_POINT('Ctrl Pts',(0.00896282356274304,-0.0414384247160302,
-0.0211386768493011));
#45399=CARTESIAN_POINT('Ctrl Pts',(0.0090086241939109,-0.0414079981827579,
-0.0210987575991451));
#45400=CARTESIAN_POINT('Ctrl Pts',(0.00909348323881466,-0.0413367207429092,
-0.0210052455063194));
#45401=CARTESIAN_POINT('Ctrl Pts',(0.00918146742562052,-0.0412396136184749,
-0.0208195277998905));
#45402=CARTESIAN_POINT('Ctrl Pts',(0.00920000311952126,-0.0411993385669761,
-0.0206824283425213));
#45403=CARTESIAN_POINT('Ctrl Pts',(0.00919999999921242,-0.0411751789487302,
-0.0206085902105018));
#45404=CARTESIAN_POINT('Ctrl Pts',(0.00898033303268563,-0.0411244170199114,
-0.0211561863192437));
#45405=CARTESIAN_POINT('Ctrl Pts',(0.0090240415983997,-0.0411163328788772,
-0.0211124767636134));
#45406=CARTESIAN_POINT('Ctrl Pts',(0.0091023983074395,-0.0410987223439349,
-0.0210124582185773));
#45407=CARTESIAN_POINT('Ctrl Pts',(0.00918085466954725,-0.0410703444398294,
-0.0208305876674043));
#45408=CARTESIAN_POINT('Ctrl Pts',(0.00920000322260556,-0.0410527962950982,
-0.0206949185075559));
#45409=CARTESIAN_POINT('Ctrl Pts',(0.0091999999991864,-0.0410443012976313,
-0.0206258213055316));
#45410=CARTESIAN_POINT('Ctrl Pts',(0.00898033008514593,-0.0409788141462712,
-0.021156183371704));
#45411=CARTESIAN_POINT('Ctrl Pts',(0.00902661141419035,-0.0409788182295161,
-0.0211099020429095));
#45412=CARTESIAN_POINT('Ctrl Pts',(0.00910698282803333,-0.0409788271246903,
-0.0210051586050165));
#45413=CARTESIAN_POINT('Ctrl Pts',(0.00918277256369496,-0.0409788414577655,
-0.0208221821890316));
#45414=CARTESIAN_POINT('Ctrl Pts',(0.00920000289980377,-0.0409788503201195,
-0.0206912792681954));
#45415=CARTESIAN_POINT('Ctrl Pts',(0.00919999999926789,-0.0409788546105533,
-0.0206258202417353));
#45416=CARTESIAN_POINT('',(0.0092,-0.040978887648424,-0.0206258532865581));
#45417=CARTESIAN_POINT('Origin',(0.00845000000001,-0.040978887648414,-0.0206258532865681));
#45418=CARTESIAN_POINT('Origin',(0.00920000000001,-0.040978887648414,-0.0198759665451198));
#45419=CARTESIAN_POINT('Origin',(0.00845,-0.0326537743898723,-0.0206258532865581));
#45420=CARTESIAN_POINT('',(0.00845,-0.0297787743898723,-0.0213758532865581));
#45421=CARTESIAN_POINT('',(0.0092,-0.0297787743898723,-0.0206258532865581));
#45422=CARTESIAN_POINT('Origin',(0.00845000000001,-0.0297787743898623,-0.0206258532865681));
#45423=CARTESIAN_POINT('',(0.00920000000001,-0.0326537743898623,-0.0206258532865681));
#45424=CARTESIAN_POINT('',(0.00845000000001,-0.0326537743898623,-0.0213758532865681));
#45425=CARTESIAN_POINT('Ctrl Pts',(-0.0157883510491121,-0.0420671792490158,
-0.0209642043356702));
#45426=CARTESIAN_POINT('Ctrl Pts',(-0.0157528254319765,-0.0420316530974381,
-0.0210352596879392));
#45427=CARTESIAN_POINT('Ctrl Pts',(-0.0156743980241011,-0.0419532255098913,
-0.0211563511198682));
#45428=CARTESIAN_POINT('Ctrl Pts',(-0.0154683058786475,-0.0417471348922467,
-0.0213244855175527));
#45429=CARTESIAN_POINT('Ctrl Pts',(-0.0153031099239451,-0.041581934857854,
-0.0213758619327538));
#45430=CARTESIAN_POINT('Ctrl Pts',(-0.0152303031410778,-0.0415091242546894,
-0.0213758532843753));
#45431=CARTESIAN_POINT('Ctrl Pts',(-0.0158238849031059,-0.0419961175614541,
-0.020999738189664));
#45432=CARTESIAN_POINT('Ctrl Pts',(-0.0157879192374373,-0.0419612102583594,
-0.0210635155071967));
#45433=CARTESIAN_POINT('Ctrl Pts',(-0.0157091531723962,-0.0418828002313692,
-0.0211749649159776));
#45434=CARTESIAN_POINT('Ctrl Pts',(-0.0155066139651694,-0.0416772361088086,
-0.0213315303341105));
#45435=CARTESIAN_POINT('Ctrl Pts',(-0.0153491317045492,-0.0415278309272449,
-0.0213758607470282));
#45436=CARTESIAN_POINT('Ctrl Pts',(-0.0152765861541394,-0.0414628494275772,
-0.0213758532846746));
#45437=CARTESIAN_POINT('Ctrl Pts',(-0.0158828479122755,-0.0418424302635563,
-0.0210587011988336));
#45438=CARTESIAN_POINT('Ctrl Pts',(-0.0158470801331243,-0.0418075947969581,
-0.0211122468869272));
#45439=CARTESIAN_POINT('Ctrl Pts',(-0.0157672464104804,-0.0417253071758865,
-0.0212106236431154));
#45440=CARTESIAN_POINT('Ctrl Pts',(-0.0155701075544912,-0.0415180843704948,
-0.021347254915059));
#45441=CARTESIAN_POINT('Ctrl Pts',(-0.0154295155527349,-0.0414081805923562,
-0.0213758581004239));
#45442=CARTESIAN_POINT('Ctrl Pts',(-0.0153569536803665,-0.0413581243643992,
-0.0213758532853428));
#45443=CARTESIAN_POINT('Ctrl Pts',(-0.0159628235627429,-0.0414384247160303,
-0.0211386768493011));
#45444=CARTESIAN_POINT('Ctrl Pts',(-0.015922904312587,-0.0414079981827581,
-0.021184477480469));
#45445=CARTESIAN_POINT('Ctrl Pts',(-0.0158293922197611,-0.0413367207429093,
-0.0212693365253728));
#45446=CARTESIAN_POINT('Ctrl Pts',(-0.0156436745133296,-0.0412396136184735,
-0.0213573207121799));
#45447=CARTESIAN_POINT('Ctrl Pts',(-0.0155065750559569,-0.0411993385669744,
-0.0213758564060802));
#45448=CARTESIAN_POINT('Ctrl Pts',(-0.0154327369239338,-0.041175178948727,
-0.0213758532857705));
#45449=CARTESIAN_POINT('Ctrl Pts',(-0.0159803330326856,-0.0411244170199117,
-0.0211561863192437));
#45450=CARTESIAN_POINT('Ctrl Pts',(-0.0159366234770553,-0.0411163328788775,
-0.0211998948849578));
#45451=CARTESIAN_POINT('Ctrl Pts',(-0.0158366049320192,-0.0410987223439351,
-0.0212782515939976));
#45452=CARTESIAN_POINT('Ctrl Pts',(-0.0156547343808434,-0.0410703444398291,
-0.0213567079561065));
#45453=CARTESIAN_POINT('Ctrl Pts',(-0.0155190652209917,-0.0410527962950975,
-0.0213758565091645));
#45454=CARTESIAN_POINT('Ctrl Pts',(-0.0154499680189642,-0.0410443012976302,
-0.0213758532857445));
#45455=CARTESIAN_POINT('Ctrl Pts',(-0.0159803300851459,-0.0409788141462715,
-0.021156183371704));
#45456=CARTESIAN_POINT('Ctrl Pts',(-0.0159340487563514,-0.0409788182295164,
-0.0212024647007484));
#45457=CARTESIAN_POINT('Ctrl Pts',(-0.0158293053184584,-0.0409788271246906,
-0.0212828361145914));
#45458=CARTESIAN_POINT('Ctrl Pts',(-0.0156463289024708,-0.0409788414577657,
-0.0213586258502542));
#45459=CARTESIAN_POINT('Ctrl Pts',(-0.0155154259816314,-0.0409788503201197,
-0.0213758561863626));
#45460=CARTESIAN_POINT('Ctrl Pts',(-0.0154499669551684,-0.0409788546105534,
-0.021375853285826));
#45461=CARTESIAN_POINT('',(-0.01545,-0.040978887648424,-0.0213758532865581));
#45462=CARTESIAN_POINT('Origin',(-0.01545000000001,-0.040978887648414,-0.0206258532865681));
#45463=CARTESIAN_POINT('Origin',(-0.0147001132585417,-0.040978887648414,
-0.0213758532865681));
#45464=CARTESIAN_POINT('Origin',(-0.01545,-0.0326537743898723,-0.0206258532865581));
#45465=CARTESIAN_POINT('',(-0.0162,-0.0297787743898723,-0.0206258532865581));
#45466=CARTESIAN_POINT('',(-0.01545,-0.0297787743898723,-0.0213758532865581));
#45467=CARTESIAN_POINT('Origin',(-0.01545000000001,-0.0297787743898623,
-0.0206258532865681));
#45468=CARTESIAN_POINT('',(-0.01545000000001,-0.0326537743898623,-0.0213758532865681));
#45469=CARTESIAN_POINT('',(-0.01620000000001,-0.0326537743898623,-0.0206258532865681));
#45470=CARTESIAN_POINT('Origin',(-0.00925,-0.0417287743898723,-0.0206258532865581));
#45471=CARTESIAN_POINT('',(-0.00924999999999,-0.0424787743898823,-0.0206258532865681));
#45472=CARTESIAN_POINT('',(-0.00924999999999,-0.0417287743898823,-0.0213758532865681));
#45473=CARTESIAN_POINT('Ctrl Pts',(0.00878840485914475,-0.0420671254389838,
-0.00338750223744656));
#45474=CARTESIAN_POINT('Ctrl Pts',(0.00875287870756701,-0.0421381807912529,
-0.00342302785458223));
#45475=CARTESIAN_POINT('Ctrl Pts',(0.00867445112002031,-0.0422592722231821,
-0.00350145526245769));
#45476=CARTESIAN_POINT('Ctrl Pts',(0.00846836050237674,-0.042427406620866,
-0.00370754740791023));
#45477=CARTESIAN_POINT('Ctrl Pts',(0.00830316046798524,-0.0424787830360672,
-0.00387274336261131));
#45478=CARTESIAN_POINT('Ctrl Pts',(0.00823034986482124,-0.0424787743876894,
-0.0039455501454778));
#45479=CARTESIAN_POINT('Ctrl Pts',(0.00871734317158272,-0.0421026592929779,
-0.00335196838345255));
#45480=CARTESIAN_POINT('Ctrl Pts',(0.00868243586848798,-0.0421664366105106,
-0.00338793404912117));
#45481=CARTESIAN_POINT('Ctrl Pts',(0.00860402584149778,-0.0422778860192916,
-0.00346670011416231));
#45482=CARTESIAN_POINT('Ctrl Pts',(0.00839846171893839,-0.0424344514374237,
-0.00366923932138805));
#45483=CARTESIAN_POINT('Ctrl Pts',(0.00824905653737574,-0.0424787818503417,
-0.00382672158200695));
#45484=CARTESIAN_POINT('Ctrl Pts',(0.00818407503770852,-0.0424787743879888,
-0.00389926713241585));
#45485=CARTESIAN_POINT('Ctrl Pts',(0.00856365587368484,-0.0421616223021476,
-0.00329300537428275));
#45486=CARTESIAN_POINT('Ctrl Pts',(0.00852882040708652,-0.0422151679902413,
-0.00332877315343396));
#45487=CARTESIAN_POINT('Ctrl Pts',(0.00844653278601497,-0.0423135447464294,
-0.00340860687607793));
#45488=CARTESIAN_POINT('Ctrl Pts',(0.00823930998062411,-0.0424501760183726,
-0.00360574573206604));
#45489=CARTESIAN_POINT('Ctrl Pts',(0.00812940620248598,-0.0424787792037377,
-0.00374633773382112));
#45490=CARTESIAN_POINT('Ctrl Pts',(0.00807934997452958,-0.042478774388657,
-0.00381889960618842));
#45491=CARTESIAN_POINT('Ctrl Pts',(0.00815965032615726,-0.0422415979526155,
-0.00321302972381497));
#45492=CARTESIAN_POINT('Ctrl Pts',(0.00812922379288498,-0.0422873985837833,
-0.00325294897397103));
#45493=CARTESIAN_POINT('Ctrl Pts',(0.00805794635303623,-0.0423722576286871,
-0.0033464610667968));
#45494=CARTESIAN_POINT('Ctrl Pts',(0.00796083922860117,-0.0424602418154937,
-0.00353217877322744));
#45495=CARTESIAN_POINT('Ctrl Pts',(0.00792056417710238,-0.0424787775093941,
-0.00366927823059887));
#45496=CARTESIAN_POINT('Ctrl Pts',(0.00789640455885557,-0.0424787743890847,
-0.00374311636262087));
#45497=CARTESIAN_POINT('Ctrl Pts',(0.00784564263003753,-0.042259107422558,
-0.00319552025387238));
#45498=CARTESIAN_POINT('Ctrl Pts',(0.00783755848900359,-0.0423028159882721,
-0.00323922980950267));
#45499=CARTESIAN_POINT('Ctrl Pts',(0.00781994795406138,-0.0423811726973118,
-0.00333924835453885));
#45500=CARTESIAN_POINT('Ctrl Pts',(0.00779157004995593,-0.0424596290594203,
-0.00352111890571367));
#45501=CARTESIAN_POINT('Ctrl Pts',(0.00777402190522475,-0.0424787776124784,
-0.00365678806556426));
#45502=CARTESIAN_POINT('Ctrl Pts',(0.00776552690775767,-0.0424787743890587,
-0.00372588526759064));
#45503=CARTESIAN_POINT('Ctrl Pts',(0.00770003975639667,-0.0422591044750182,
-0.00319552320141217));
#45504=CARTESIAN_POINT('Ctrl Pts',(0.00770004383964169,-0.0423053858040628,
-0.00324180453020672));
#45505=CARTESIAN_POINT('Ctrl Pts',(0.00770005273481624,-0.0423857572179058,
-0.00334654796809979));
#45506=CARTESIAN_POINT('Ctrl Pts',(0.00770006706789182,-0.042461546953568,
-0.00352952438408646));
#45507=CARTESIAN_POINT('Ctrl Pts',(0.00770007593024613,-0.0424787772896766,
-0.00366042730492475));
#45508=CARTESIAN_POINT('Ctrl Pts',(0.00770008022067997,-0.0424787743891402,
-0.00372588633138674));
#45509=CARTESIAN_POINT('',(0.0077001132585517,-0.0424787743898723,-0.00372585328655811));
#45510=CARTESIAN_POINT('Origin',(0.0077001132585617,-0.0417287743898823,
-0.00372585328654811));
#45511=CARTESIAN_POINT('Origin',(0.0077001132585617,-0.0424787743898823,
-0.00447574002801644));
#45512=CARTESIAN_POINT('Origin',(0.00845,-0.0355287743470315,-0.00372585328655811));
#45513=CARTESIAN_POINT('',(0.0092,-0.0297787743898723,-0.0037258532865581));
#45514=CARTESIAN_POINT('',(0.00845,-0.0297787743898723,-0.0029758532865581));
#45515=CARTESIAN_POINT('Origin',(0.00845000000001,-0.0297787743898623,-0.0037258532865481));
#45516=CARTESIAN_POINT('',(0.00845000000001,-0.0355287743470215,-0.0029758532865481));
#45517=CARTESIAN_POINT('',(0.00920000000001,-0.0355287743470215,-0.00372585328654811));
#45518=CARTESIAN_POINT('Ctrl Pts',(-0.0157884048591435,-0.0420671254389844,
-0.00338750223744594));
#45519=CARTESIAN_POINT('Ctrl Pts',(-0.0157528787075658,-0.0420315998218488,
-0.00331644688517705));
#45520=CARTESIAN_POINT('Ctrl Pts',(-0.0156744511200191,-0.0419531724139733,
-0.00319535545324795));
#45521=CARTESIAN_POINT('Ctrl Pts',(-0.0154683605023745,-0.0417470802685198,
-0.00302722105556351));
#45522=CARTESIAN_POINT('Ctrl Pts',(-0.0153031604679818,-0.0415818843138174,
-0.00297584464036245));
#45523=CARTESIAN_POINT('Ctrl Pts',(-0.0152303498648171,-0.0415090775309501,
-0.00297585328874096));
#45524=CARTESIAN_POINT('Ctrl Pts',(-0.0157173431715818,-0.0421026592929782,
-0.00335196838345221));
#45525=CARTESIAN_POINT('Ctrl Pts',(-0.0156824358684872,-0.0420666936273096,
-0.00328819106591947));
#45526=CARTESIAN_POINT('Ctrl Pts',(-0.0156040258414969,-0.0419879275622684,
-0.00317674165713853));
#45527=CARTESIAN_POINT('Ctrl Pts',(-0.0153984617189363,-0.0417853883550417,
-0.00302017623900573));
#45528=CARTESIAN_POINT('Ctrl Pts',(-0.0152490565373728,-0.0416279060944215,
-0.002975845826088));
#45529=CARTESIAN_POINT('Ctrl Pts',(-0.0151840750377049,-0.0415553605440117,
-0.00297585328844161));
#45530=CARTESIAN_POINT('Ctrl Pts',(-0.0155636558736841,-0.0421616223021478,
-0.0032930053742826));
#45531=CARTESIAN_POINT('Ctrl Pts',(-0.0155288204070858,-0.0421258545229966,
-0.00323945968618904));
#45532=CARTESIAN_POINT('Ctrl Pts',(-0.0154465327860142,-0.0420460208003526,
-0.00314108293000091));
#45533=CARTESIAN_POINT('Ctrl Pts',(-0.0152393099806225,-0.0418488819443635,
-0.00300445165805714));
#45534=CARTESIAN_POINT('Ctrl Pts',(-0.0151294062024839,-0.0417082899426073,
-0.00297584847269226));
#45535=CARTESIAN_POINT('Ctrl Pts',(-0.0150793499745268,-0.0416357280702388,
-0.00297585328777345));
#45536=CARTESIAN_POINT('Ctrl Pts',(-0.015159650326158,-0.0422415979526153,
-0.00321302972381513));
#45537=CARTESIAN_POINT('Ctrl Pts',(-0.0151292237928857,-0.0422016787024593,
-0.00316722909264727));
#45538=CARTESIAN_POINT('Ctrl Pts',(-0.015057946353037,-0.0421081666096335,
-0.00308237004774347));
#45539=CARTESIAN_POINT('Ctrl Pts',(-0.0149608392286012,-0.0419224489032019,
-0.00299438586093631));
#45540=CARTESIAN_POINT('Ctrl Pts',(-0.0149205641771022,-0.0417853494458292,
-0.00297585016703602));
#45541=CARTESIAN_POINT('Ctrl Pts',(-0.0148964045588548,-0.041711511313806,
-0.00297585328734569));
#45542=CARTESIAN_POINT('Ctrl Pts',(-0.0148456426300393,-0.0422591074225579,
-0.00319552025387248));
#45543=CARTESIAN_POINT('Ctrl Pts',(-0.0148375584890053,-0.0422153978669277,
-0.00315181168815843));
#45544=CARTESIAN_POINT('Ctrl Pts',(-0.0148199479540628,-0.0421153793218916,
-0.00307345497911859));
#45545=CARTESIAN_POINT('Ctrl Pts',(-0.0147915700499568,-0.0419335087707158,
-0.00299499861700968));
#45546=CARTESIAN_POINT('Ctrl Pts',(-0.0147740219052253,-0.041797839610864,
-0.00297585006395169));
#45547=CARTESIAN_POINT('Ctrl Pts',(-0.014765526907758,-0.0417287424088365,
-0.00297585328737171));
#45548=CARTESIAN_POINT('Ctrl Pts',(-0.0147000397563992,-0.0422591044750182,
-0.00319552320141217));
#45549=CARTESIAN_POINT('Ctrl Pts',(-0.0147000438396441,-0.0422128231462237,
-0.00314924187236774));
#45550=CARTESIAN_POINT('Ctrl Pts',(-0.0147000527348183,-0.0421080797083307,
-0.00306887045852474));
#45551=CARTESIAN_POINT('Ctrl Pts',(-0.0147000670678934,-0.0419251032923432,
-0.002993080722862));
#45552=CARTESIAN_POINT('Ctrl Pts',(-0.0147000759302474,-0.0417942003715037,
-0.00297585038675357));
#45553=CARTESIAN_POINT('Ctrl Pts',(-0.0147000802206811,-0.0417287413450406,
-0.00297585328729021));
#45554=CARTESIAN_POINT('',(-0.0147001132585517,-0.0417287743898723,-0.00297585328655811));
#45555=CARTESIAN_POINT('Origin',(-0.0147001132585417,-0.0417287743898823,
-0.00372585328654811));
#45556=CARTESIAN_POINT('Origin',(-0.0147001132585417,-0.040978887648414,
-0.00297585328654811));
#45557=CARTESIAN_POINT('Origin',(-0.01545,-0.0355287743470315,-0.00372585328655811));
#45558=CARTESIAN_POINT('',(-0.01545,-0.0297787743898723,-0.0029758532865581));
#45559=CARTESIAN_POINT('',(-0.0162,-0.0297787743898723,-0.0037258532865581));
#45560=CARTESIAN_POINT('Origin',(-0.01545000000001,-0.0297787743898623,
-0.0037258532865481));
#45561=CARTESIAN_POINT('',(-0.01620000000001,-0.0355287743470215,-0.00372585328654811));
#45562=CARTESIAN_POINT('',(-0.01545000000001,-0.0355287743470215,-0.0029758532865481));
#45563=CARTESIAN_POINT('Origin',(-0.01545,-0.0417287743898723,-0.0121758532865581));
#45564=CARTESIAN_POINT('',(-0.01545000000001,-0.0424787743898823,-0.0121758532865681));
#45565=CARTESIAN_POINT('',(-0.01620000000001,-0.0417287743898823,-0.0121758532865681));
#45566=CARTESIAN_POINT('Origin',(-0.0035,-0.0417287743898723,-0.00372585328655811));
#45567=CARTESIAN_POINT('',(-0.00349999999999,-0.0424787743898823,-0.00372585328654811));
#45568=CARTESIAN_POINT('',(-0.00349999999999,-0.0417287743898823,-0.00297585328654811));
#45569=CARTESIAN_POINT('Origin',(0.00845,-0.0417287743898723,-0.0121758532865581));
#45570=CARTESIAN_POINT('',(0.00845000000001,-0.0424787743898823,-0.0121758532865681));
#45571=CARTESIAN_POINT('',(0.00920000000001,-0.0417287743898823,-0.0121758532865681));
#45572=CARTESIAN_POINT('Origin',(-0.015,-0.0297787743898723,-0.0213758532865581));
#45573=CARTESIAN_POINT('',(-0.0095,-0.0297787743898723,-0.0213758532865581));
#45574=CARTESIAN_POINT('',(-0.015,-0.0297787743898623,-0.0213758532865681));
#45575=CARTESIAN_POINT('',(-0.0095,-0.0372787743898723,-0.0213758532865581));
#45576=CARTESIAN_POINT('',(-0.00949999999999,-0.0372787743898623,-0.0213758532865681));
#45577=CARTESIAN_POINT('',(-0.0035,-0.0372787743898723,-0.0213758532865581));
#45578=CARTESIAN_POINT('Origin',(-0.00649999999999,-0.0372787743898623,
-0.0213758532865681));
#45579=CARTESIAN_POINT('',(-0.0035,-0.0285787743898723,-0.0213758532865581));
#45580=CARTESIAN_POINT('',(-0.00349999999999,-0.0372787743898623,-0.0213758532865681));
#45581=CARTESIAN_POINT('',(0.0045,-0.0285787743898723,-0.0213758532865581));
#45582=CARTESIAN_POINT('',(0.00450000000001,-0.0285787743898623,-0.0213758532865681));
#45583=CARTESIAN_POINT('',(0.0045,-0.035138261906077,-0.0213758532865581));
#45584=CARTESIAN_POINT('',(0.00450000000001,-0.0297787743898623,-0.0213758532865681));
#45585=CARTESIAN_POINT('',(0.0075,-0.035138261906077,-0.0213758532865581));
#45586=CARTESIAN_POINT('Origin',(0.00600000000001,-0.0355287743898623,-0.0213758532865681));
#45587=CARTESIAN_POINT('',(0.0075,-0.0297787743898723,-0.0213758532865581));
#45588=CARTESIAN_POINT('',(0.00750000000001,-0.0355287743898623,-0.0213758532865681));
#45589=CARTESIAN_POINT('',(-0.015,-0.0297787743898623,-0.0213758532865681));
#45590=CARTESIAN_POINT('Origin',(-0.0095,-0.0297787743898723,-0.0041758532865581));
#45591=CARTESIAN_POINT('',(-0.0162,-0.0297787743898723,-0.0189258532865581));
#45592=CARTESIAN_POINT('',(-0.01620000000001,-0.0297787743898623,-0.0213758532865681));
#45593=CARTESIAN_POINT('',(-0.015,-0.0297787743898723,-0.0189258532865581));
#45594=CARTESIAN_POINT('',(-0.01119999999999,-0.0297787743898623,-0.0189258532865681));
#45595=CARTESIAN_POINT('',(-0.015,-0.0297787743898723,-0.0201758532865581));
#45596=CARTESIAN_POINT('',(-0.015,-0.0297787743898623,-0.0213758532865681));
#45597=CARTESIAN_POINT('',(-0.0095,-0.0297787743898723,-0.0201758532865581));
#45598=CARTESIAN_POINT('',(-0.00924999999999,-0.0297787743898623,-0.0201758532865681));
#45599=CARTESIAN_POINT('',(-0.00949999999999,-0.0297787743898623,-0.0029758532865481));
#45600=CARTESIAN_POINT('Origin',(-0.0162,-0.0355287743898723,-0.0121758532865581));
#45601=CARTESIAN_POINT('',(-0.0162,-0.0297787743898723,-0.0054258532865581));
#45602=CARTESIAN_POINT('',(-0.01620000000001,-0.0297787743898623,-0.0213758532865681));
#45603=CARTESIAN_POINT('',(-0.0162,-0.0285787743898723,-0.0054258532865581));
#45604=CARTESIAN_POINT('',(-0.01620000000001,-0.0297787743898623,-0.0054258532865681));
#45605=CARTESIAN_POINT('',(-0.0162,-0.0285787743898723,-0.0104258532865581));
#45606=CARTESIAN_POINT('',(-0.01620000000001,-0.0285787743898623,-0.0104258532865681));
#45607=CARTESIAN_POINT('',(-0.0162,-0.0297787743898723,-0.0104258532865581));
#45608=CARTESIAN_POINT('',(-0.01620000000001,-0.0297787743898623,-0.0104258532865681));
#45609=CARTESIAN_POINT('',(-0.0162,-0.0297787743898723,-0.0139258532865581));
#45610=CARTESIAN_POINT('',(-0.01620000000001,-0.0297787743898623,-0.0213758532865681));
#45611=CARTESIAN_POINT('',(-0.0162,-0.0285787743898723,-0.0139258532865581));
#45612=CARTESIAN_POINT('',(-0.01620000000001,-0.0297787743898623,-0.0139258532865681));
#45613=CARTESIAN_POINT('',(-0.0162,-0.0285787743898723,-0.0189258532865581));
#45614=CARTESIAN_POINT('',(-0.01620000000001,-0.0285787743898623,-0.0139258532865681));
#45615=CARTESIAN_POINT('',(-0.01620000000001,-0.0297787743898623,-0.0189258532865681));
#45616=CARTESIAN_POINT('Origin',(-0.0095,-0.0297787743898723,-0.0041758532865581));
#45617=CARTESIAN_POINT('',(-0.0095,-0.0297787743898723,-0.0029758532865581));
#45618=CARTESIAN_POINT('',(-0.015,-0.0297787743898623,-0.0029758532865481));
#45619=CARTESIAN_POINT('',(-0.0095,-0.0297787743898723,-0.0041758532865581));
#45620=CARTESIAN_POINT('',(-0.00949999999999,-0.0297787743898623,-0.0041758532865581));
#45621=CARTESIAN_POINT('',(-0.015,-0.0297787743898723,-0.0041758532865581));
#45622=CARTESIAN_POINT('',(-0.015,-0.0297787743898623,-0.0041758532865581));
#45623=CARTESIAN_POINT('',(-0.015,-0.0297787743898723,-0.0054258532865581));
#45624=CARTESIAN_POINT('',(-0.015,-0.0297787743898623,-0.0213758532865681));
#45625=CARTESIAN_POINT('',(-0.01284999999999,-0.0297787743898623,-0.0054258532865681));
#45626=CARTESIAN_POINT('Origin',(-0.0035,-0.0424787743898723,-0.0121758532865581));
#45627=CARTESIAN_POINT('',(-0.00685,-0.0424787743898823,-0.0121758532865581));
#45628=CARTESIAN_POINT('Origin',(1.00006808390063E-14,-0.0424787743898823,
-0.0121758532865681));
#45629=CARTESIAN_POINT('',(-0.015,-0.0424787743898823,-0.0121758532865581));
#45630=CARTESIAN_POINT('Origin',(-0.01249999999999,-0.0424787743898823,
-0.0121758532865681));
#45631=CARTESIAN_POINT('Origin',(-0.0139,-0.0295787743898723,-0.0066758532865581));
#45632=CARTESIAN_POINT('',(-0.0129,-0.0295787743898723,-0.0104258532865581));
#45633=CARTESIAN_POINT('',(-0.0139,-0.0285787743898723,-0.0104258532865581));
#45634=CARTESIAN_POINT('Origin',(-0.01389999999999,-0.0295787743898623,
-0.0104258532865681));
#45635=CARTESIAN_POINT('',(-0.0139,-0.0285787743898723,-0.0054258532865581));
#45636=CARTESIAN_POINT('',(-0.01389999999999,-0.0285787743898623,-0.0066758532865681));
#45637=CARTESIAN_POINT('',(-0.0129,-0.0295787743898723,-0.0054258532865581));
#45638=CARTESIAN_POINT('Origin',(-0.01389999999999,-0.0295787743898623,
-0.0054258532865681));
#45639=CARTESIAN_POINT('',(-0.01289999999999,-0.0295787743898623,-0.0066758532865681));
#45640=CARTESIAN_POINT('Origin',(-0.01455,-0.0285787743898723,-0.0079258532865581));
#45641=CARTESIAN_POINT('',(-0.01289999999999,-0.0285787743898623,-0.0104258532865681));
#45642=CARTESIAN_POINT('',(-0.01620000000001,-0.0285787743898623,-0.0054258532865681));
#45643=CARTESIAN_POINT('Origin',(-0.0129,-0.0297787743898723,-0.0104258532865581));
#45644=CARTESIAN_POINT('',(-0.0129,-0.0297787743898723,-0.0104258532865581));
#45645=CARTESIAN_POINT('',(-0.01289999999999,-0.0297787743898623,-0.0104258532865681));
#45646=CARTESIAN_POINT('',(-0.015,-0.0297787743898723,-0.0104258532865581));
#45647=CARTESIAN_POINT('',(-0.01289999999999,-0.0297787743898623,-0.0104258532865681));
#45648=CARTESIAN_POINT('',(-0.01119999999999,-0.0297787743898623,-0.0104258532865681));
#45649=CARTESIAN_POINT('Origin',(-0.0139,-0.0295787743898723,-0.0151758532865581));
#45650=CARTESIAN_POINT('',(-0.0129,-0.0295787743898723,-0.0189258532865581));
#45651=CARTESIAN_POINT('',(-0.0139,-0.0285787743898723,-0.0189258532865581));
#45652=CARTESIAN_POINT('Origin',(-0.01389999999999,-0.0295787743898623,
-0.0189258532865681));
#45653=CARTESIAN_POINT('',(-0.0139,-0.0285787743898723,-0.0139258532865581));
#45654=CARTESIAN_POINT('',(-0.01389999999999,-0.0285787743898623,-0.0151758532865681));
#45655=CARTESIAN_POINT('',(-0.0129,-0.0295787743898723,-0.0139258532865581));
#45656=CARTESIAN_POINT('Origin',(-0.01389999999999,-0.0295787743898623,
-0.0139258532865681));
#45657=CARTESIAN_POINT('',(-0.01289999999999,-0.0295787743898623,-0.0151758532865681));
#45658=CARTESIAN_POINT('Origin',(-0.01455,-0.0285787743898723,-0.0164258532865581));
#45659=CARTESIAN_POINT('',(-0.01620000000001,-0.0285787743898623,-0.0189258532865681));
#45660=CARTESIAN_POINT('',(-0.01289999999999,-0.0285787743898623,-0.0139258532865681));
#45661=CARTESIAN_POINT('Origin',(-0.0129,-0.0297787743898723,-0.0189258532865581));
#45662=CARTESIAN_POINT('',(-0.0129,-0.0297787743898723,-0.0189258532865581));
#45663=CARTESIAN_POINT('',(-0.01289999999999,-0.0297787743898623,-0.0189258532865681));
#45664=CARTESIAN_POINT('',(-0.01620000000001,-0.0297787743898623,-0.0189258532865681));
#45665=CARTESIAN_POINT('Origin',(-0.0015,-0.0295787743898723,-0.0190758532865581));
#45666=CARTESIAN_POINT('',(0.0045,-0.0295787743898723,-0.0180758532865581));
#45667=CARTESIAN_POINT('',(0.0045,-0.0285787743898723,-0.0190758532865581));
#45668=CARTESIAN_POINT('Origin',(0.00450000000001,-0.0295787743898623,-0.0190758532865681));
#45669=CARTESIAN_POINT('',(-0.0035,-0.0285787743898723,-0.0190758532865581));
#45670=CARTESIAN_POINT('',(-0.00149999999999,-0.0285787743898623,-0.0190758532865681));
#45671=CARTESIAN_POINT('',(-0.0035,-0.0295787743898723,-0.0180758532865581));
#45672=CARTESIAN_POINT('Origin',(-0.00349999999999,-0.0295787743898623,
-0.0190758532865681));
#45673=CARTESIAN_POINT('',(-0.00149999999999,-0.0295787743898623,-0.0180758532865681));
#45674=CARTESIAN_POINT('Origin',(-0.0035,-0.0372787743898723,-0.00297585328655811));
#45675=CARTESIAN_POINT('',(-0.00349999999999,-0.0285787743898623,-0.0213758532865681));
#45676=CARTESIAN_POINT('',(-0.0035,-0.0372787743898723,-0.0201758532865581));
#45677=CARTESIAN_POINT('',(-0.00349999999999,-0.0372787743898623,-0.0029758532865481));
#45678=CARTESIAN_POINT('',(-0.0035,-0.0297787743898723,-0.0201758532865581));
#45679=CARTESIAN_POINT('',(-0.00349999999999,-0.0364037743470214,-0.0201758532865681));
#45680=CARTESIAN_POINT('',(-0.0035,-0.0297787743898723,-0.0180758532865581));
#45681=CARTESIAN_POINT('',(-0.00349999999999,-0.0297787743898623,-0.0213758532865681));
#45682=CARTESIAN_POINT('',(-0.00349999999999,-0.0297787743898623,-0.0180758532865681));
#45683=CARTESIAN_POINT('Origin',(0.0005,-0.0285787743898723,-0.0197258532865581));
#45684=CARTESIAN_POINT('',(0.00450000000001,-0.0285787743898623,-0.0180758532865681));
#45685=CARTESIAN_POINT('Origin',(0.0025,-0.0295787743898723,-0.0052758532865581));
#45686=CARTESIAN_POINT('',(-0.0035,-0.0295787743898723,-0.0062758532865581));
#45687=CARTESIAN_POINT('',(-0.0035,-0.0285787743898723,-0.0052758532865581));
#45688=CARTESIAN_POINT('Origin',(-0.00349999999999,-0.0295787743898623,
-0.0052758532865681));
#45689=CARTESIAN_POINT('',(0.0045,-0.0285787743898723,-0.0052758532865581));
#45690=CARTESIAN_POINT('',(0.00250000000001,-0.0285787743898623,-0.0052758532865681));
#45691=CARTESIAN_POINT('',(0.0045,-0.0295787743898723,-0.0062758532865581));
#45692=CARTESIAN_POINT('Origin',(0.00450000000001,-0.0295787743898623,-0.0052758532865681));
#45693=CARTESIAN_POINT('',(0.00250000000001,-0.0295787743898623,-0.0062758532865681));
#45694=CARTESIAN_POINT('Origin',(0.0045,-0.035138261906077,-0.0041758532865581));
#45695=CARTESIAN_POINT('',(0.0045,-0.0285787743898723,-0.0029758532865581));
#45696=CARTESIAN_POINT('',(0.00450000000001,-0.0285787743898623,-0.0062758532865681));
#45697=CARTESIAN_POINT('',(0.0045,-0.035138261906077,-0.00297585328655811));
#45698=CARTESIAN_POINT('',(0.00450000000001,-0.0355287743898623,-0.0029758532865481));
#45699=CARTESIAN_POINT('',(0.0045,-0.035138261906077,-0.0041758532865581));
#45700=CARTESIAN_POINT('',(0.00450000000001,-0.035138261906067,-0.0041758532865581));
#45701=CARTESIAN_POINT('',(0.0045,-0.0297787743898723,-0.0041758532865581));
#45702=CARTESIAN_POINT('',(0.00450000000001,-0.0355287743898623,-0.0041758532865581));
#45703=CARTESIAN_POINT('',(0.0045,-0.0297787743898723,-0.0062758532865581));
#45704=CARTESIAN_POINT('',(0.00450000000001,-0.0297787743898623,-0.0062758532865681));
#45705=CARTESIAN_POINT('',(0.00450000000001,-0.0297787743898623,-0.0062758532865681));
#45706=CARTESIAN_POINT('Origin',(0.0005,-0.0285787743898723,-0.0046258532865581));
#45707=CARTESIAN_POINT('',(-0.0035,-0.0285787743898723,-0.0029758532865581));
#45708=CARTESIAN_POINT('',(-0.00349999999999,-0.0285787743898623,-0.00297585328654809));
#45709=CARTESIAN_POINT('',(0.00450000000001,-0.0285787743898623,-0.00297585328654809));
#45710=CARTESIAN_POINT('Origin',(0.0069,-0.0295787743898723,-0.0155508532865581));
#45711=CARTESIAN_POINT('',(0.0059,-0.0295787743898723,-0.0054258532865581));
#45712=CARTESIAN_POINT('',(0.0069,-0.0285787743898723,-0.0054258532865581));
#45713=CARTESIAN_POINT('Origin',(0.00690000000001,-0.0295787743898623,-0.0054258532865681));
#45714=CARTESIAN_POINT('',(0.0069,-0.0285787743898723,-0.0189258532865581));
#45715=CARTESIAN_POINT('',(0.00690000000001,-0.0285787743898623,-0.0155508532865681));
#45716=CARTESIAN_POINT('',(0.0059,-0.0295787743898723,-0.0189258532865581));
#45717=CARTESIAN_POINT('Origin',(0.00690000000001,-0.0295787743898623,-0.0189258532865681));
#45718=CARTESIAN_POINT('',(0.00590000000001,-0.0295787743898623,-0.0155508532865681));
#45719=CARTESIAN_POINT('Origin',(0.00755,-0.0285787743898723,-0.0121758532865581));
#45720=CARTESIAN_POINT('',(0.0092,-0.0285787743898723,-0.0054258532865581));
#45721=CARTESIAN_POINT('',(0.00920000000001,-0.0285787743898623,-0.0054258532865681));
#45722=CARTESIAN_POINT('',(0.0092,-0.0285787743898723,-0.0189258532865581));
#45723=CARTESIAN_POINT('',(0.00920000000001,-0.0285787743898623,-0.0189258532865681));
#45724=CARTESIAN_POINT('',(0.00590000000001,-0.0285787743898623,-0.0189258532865681));
#45725=CARTESIAN_POINT('Origin',(0.0059,-0.0297787743898723,-0.0054258532865581));
#45726=CARTESIAN_POINT('',(0.0059,-0.0297787743898723,-0.0054258532865581));
#45727=CARTESIAN_POINT('',(0.00590000000001,-0.0297787743898623,-0.0054258532865681));
#45728=CARTESIAN_POINT('',(0.008,-0.0297787743898723,-0.0054258532865581));
#45729=CARTESIAN_POINT('',(0.00920000000001,-0.0297787743898623,-0.0054258532865681));
#45730=CARTESIAN_POINT('',(0.0092,-0.0297787743898723,-0.0054258532865581));
#45731=CARTESIAN_POINT('',(0.00695000000001,-0.0297787743898623,-0.0054258532865681));
#45732=CARTESIAN_POINT('',(0.00920000000001,-0.0297787743898623,-0.0054258532865681));
#45733=CARTESIAN_POINT('Origin',(0.00755,-0.0297787743898723,-0.0121758532865581));
#45734=CARTESIAN_POINT('',(0.008,-0.0297787743898723,-0.0189258532865581));
#45735=CARTESIAN_POINT('',(0.00800000000001,-0.0297787743898623,-0.0029758532865481));
#45736=CARTESIAN_POINT('',(0.0059,-0.0297787743898723,-0.0189258532865581));
#45737=CARTESIAN_POINT('',(0.00590000000001,-0.0297787743898623,-0.0054258532865681));
#45738=CARTESIAN_POINT('',(0.00590000000001,-0.0297787743898623,-0.0189258532865681));
#45739=CARTESIAN_POINT('Origin',(0.0059,-0.0297787743898723,-0.0189258532865581));
#45740=CARTESIAN_POINT('',(0.00590000000001,-0.0297787743898623,-0.0189258532865681));
#45741=CARTESIAN_POINT('Origin',(0.0092,-0.0297787743898723,-0.0189258532865581));
#45742=CARTESIAN_POINT('',(0.0092,-0.0297787743898723,-0.0189258532865581));
#45743=CARTESIAN_POINT('',(0.00920000000001,-0.0297787743898623,-0.0189258532865681));
#45744=CARTESIAN_POINT('',(0.00860000000001,-0.0297787743898623,-0.0189258532865681));
#45745=CARTESIAN_POINT('Origin',(0.008,-0.0297787743898723,-0.0041758532865581));
#45746=CARTESIAN_POINT('',(0.00920000000001,-0.0297787743898623,-0.0029758532865481));
#45747=CARTESIAN_POINT('',(0.008,-0.0297787743898723,-0.0041758532865581));
#45748=CARTESIAN_POINT('',(0.00800000000001,-0.0297787743898623,-0.0029758532865481));
#45749=CARTESIAN_POINT('',(0.0075,-0.0297787743898723,-0.0041758532865581));
#45750=CARTESIAN_POINT('',(-0.015,-0.0297787743898623,-0.0041758532865581));
#45751=CARTESIAN_POINT('',(0.0075,-0.0297787743898723,-0.0029758532865581));
#45752=CARTESIAN_POINT('',(0.00750000000001,-0.0297787743898623,-0.0041758532865581));
#45753=CARTESIAN_POINT('',(0.00800000000001,-0.0297787743898623,-0.0029758532865481));
#45754=CARTESIAN_POINT('Origin',(0.008,-0.0297787743898723,-0.0041758532865581));
#45755=CARTESIAN_POINT('',(0.0075,-0.0297787743898723,-0.0201758532865581));
#45756=CARTESIAN_POINT('',(0.00750000000001,-0.0297787743898623,-0.0029758532865481));
#45757=CARTESIAN_POINT('',(0.008,-0.0297787743898723,-0.0201758532865581));
#45758=CARTESIAN_POINT('',(0.00200000000001,-0.0297787743898623,-0.0201758532865681));
#45759=CARTESIAN_POINT('',(0.00800000000001,-0.0297787743898623,-0.0029758532865481));
#45760=CARTESIAN_POINT('',(0.00920000000001,-0.0297787743898623,-0.0029758532865481));
#45761=CARTESIAN_POINT('Origin',(-0.0129,-0.0297787743898723,-0.0054258532865581));
#45762=CARTESIAN_POINT('',(-0.0129,-0.0297787743898723,-0.0054258532865581));
#45763=CARTESIAN_POINT('',(-0.01289999999999,-0.0297787743898623,-0.0054258532865681));
#45764=CARTESIAN_POINT('',(-0.01289999999999,-0.0297787743898623,-0.0054258532865681));
#45765=CARTESIAN_POINT('Origin',(-0.0162,-0.0297787743898723,-0.0054258532865581));
#45766=CARTESIAN_POINT('',(-0.01620000000001,-0.0297787743898623,-0.0054258532865681));
#45767=CARTESIAN_POINT('Origin',(-0.01455,-0.0297787743898723,-0.0079258532865581));
#45768=CARTESIAN_POINT('',(-0.015,-0.0297787743898623,-0.0213758532865681));
#45769=CARTESIAN_POINT('Origin',(-0.0095,-0.0297787743898723,-0.0041758532865581));
#45770=CARTESIAN_POINT('',(-0.015,-0.0297787743898723,-0.0139258532865581));
#45771=CARTESIAN_POINT('',(-0.015,-0.0297787743898623,-0.0213758532865681));
#45772=CARTESIAN_POINT('',(-0.01284999999999,-0.0297787743898623,-0.0139258532865681));
#45773=CARTESIAN_POINT('Origin',(0.0045,-0.0297787743898723,-0.0062758532865581));
#45774=CARTESIAN_POINT('',(-0.0035,-0.0297787743898723,-0.0062758532865581));
#45775=CARTESIAN_POINT('',(-0.00349999999999,-0.0297787743898623,-0.0062758532865681));
#45776=CARTESIAN_POINT('',(-0.00349999999999,-0.0297787743898623,-0.0062758532865681));
#45777=CARTESIAN_POINT('Origin',(0.0005,-0.0297787743898723,-0.0046258532865581));
#45778=CARTESIAN_POINT('',(-0.0035,-0.0297787743898723,-0.0041758532865581));
#45779=CARTESIAN_POINT('',(-0.015,-0.0297787743898623,-0.0041758532865581));
#45780=CARTESIAN_POINT('',(-0.00349999999999,-0.0297787743898623,-0.0029758532865481));
#45781=CARTESIAN_POINT('Origin',(-0.01455,-0.0297787743898723,-0.0164258532865581));
#45782=CARTESIAN_POINT('',(-0.015,-0.0297787743898623,-0.0213758532865681));
#45783=CARTESIAN_POINT('',(-0.0129,-0.0297787743898723,-0.0139258532865581));
#45784=CARTESIAN_POINT('',(-0.01289999999999,-0.0297787743898623,-0.0189258532865681));
#45785=CARTESIAN_POINT('',(-0.01289999999999,-0.0297787743898623,-0.0139258532865681));
#45786=CARTESIAN_POINT('Origin',(-0.0129,-0.0297787743898723,-0.0139258532865581));
#45787=CARTESIAN_POINT('',(-0.01289999999999,-0.0297787743898623,-0.0139258532865681));
#45788=CARTESIAN_POINT('Origin',(-0.0162,-0.0297787743898723,-0.0139258532865581));
#45789=CARTESIAN_POINT('Origin',(-0.0035,-0.0297787743898723,-0.0180758532865581));
#45790=CARTESIAN_POINT('',(0.0045,-0.0297787743898723,-0.0180758532865581));
#45791=CARTESIAN_POINT('',(-0.00349999999999,-0.0297787743898623,-0.0180758532865681));
#45792=CARTESIAN_POINT('',(0.00450000000001,-0.0297787743898623,-0.0180758532865681));
#45793=CARTESIAN_POINT('Origin',(0.0005,-0.0297787743898723,-0.0197258532865581));
#45794=CARTESIAN_POINT('',(0.0045,-0.0297787743898723,-0.0201758532865581));
#45795=CARTESIAN_POINT('',(-0.00349999999999,-0.0297787743898623,-0.0201758532865681));
#45796=CARTESIAN_POINT('',(0.00450000000001,-0.0297787743898623,-0.0180758532865681));
#45797=CARTESIAN_POINT('Origin',(0.,-0.0440787743898723,-0.0121758532865581));
#45798=CARTESIAN_POINT('',(-0.00525,-0.0440787743898823,-0.0121758532865581));
#45799=CARTESIAN_POINT('Origin',(-0.00685,-0.0440787743898723,-0.0121758532865581));
#45800=CARTESIAN_POINT('Origin',(1.00006808390063E-14,-0.0440787743898823,
-0.0121758532865681));
#45801=CARTESIAN_POINT('Origin',(0.,-0.0412787743898723,-0.0121758532865581));
#45802=CARTESIAN_POINT('',(-0.0041,-0.0412787743898723,-0.0121758532865581));
#45803=CARTESIAN_POINT('Origin',(1.00006808390063E-14,-0.0412787743898723,
-0.0121758532865681));
#45804=CARTESIAN_POINT('',(-0.0041,-0.0440787743898823,-0.0121758532865581));
#45805=CARTESIAN_POINT('',(-0.0041,-0.0412787743898723,-0.0121758532865581));
#45806=CARTESIAN_POINT('Origin',(1.00006808390063E-14,-0.0440787743898823,
-0.0121758532865681));
#45807=CARTESIAN_POINT('Origin',(0.,-0.0440787743898723,-0.0121758532865581));
#45808=CARTESIAN_POINT('Origin',(-0.0035,-0.0412787743898723,-0.0121758532865581));
#45809=CARTESIAN_POINT('',(-0.015,-0.0412787743898723,-0.0121758532865581));
#45810=CARTESIAN_POINT('Origin',(-0.01249999999999,-0.0412787743898723,
-0.0121758532865681));
#45811=CARTESIAN_POINT('',(-0.015,-0.0412787743898723,-0.00417585328655811));
#45812=CARTESIAN_POINT('',(-0.015,-0.0412787743898723,-0.00297585328654811));
#45813=CARTESIAN_POINT('',(0.008,-0.0412787743898723,-0.00417585328655811));
#45814=CARTESIAN_POINT('',(0.00800000000001,-0.0412787743898723,-0.00417585328655811));
#45815=CARTESIAN_POINT('',(0.008,-0.0412787743898723,-0.0201758532865581));
#45816=CARTESIAN_POINT('',(0.00800000000001,-0.0412787743898723,-0.0213758532865681));
#45817=CARTESIAN_POINT('',(-0.015,-0.0412787743898723,-0.0201758532865581));
#45818=CARTESIAN_POINT('',(0.00225000000001,-0.0412787743898723,-0.0201758532865681));
#45819=CARTESIAN_POINT('',(-0.015,-0.0412787743898723,-0.00297585328654811));
#45820=CARTESIAN_POINT('Origin',(-0.0125,-0.0412787743898723,-0.0121758532865581));
#45821=CARTESIAN_POINT('',(-0.015,-0.0412787743898723,-0.0121758532865581));
#45822=CARTESIAN_POINT('Origin',(0.008,-0.0355287743898723,-0.0121758532865581));
#45823=CARTESIAN_POINT('',(0.00800000000001,-0.0297787743898623,-0.0041758532865581));
#45824=CARTESIAN_POINT('',(0.00800000000001,-0.0326537743470214,-0.0201758532865681));
#45825=CARTESIAN_POINT('Origin',(0.0092,-0.0355287743898723,-0.0121758532865581));
#45826=CARTESIAN_POINT('Origin',(-0.0035,-0.0355287743041906,-0.0201758532865581));
#45827=CARTESIAN_POINT('',(0.0045,-0.035138261906077,-0.0201758532865581));
#45828=CARTESIAN_POINT('',(0.00450000000001,-0.0326537743470214,-0.0201758532865681));
#45829=CARTESIAN_POINT('',(-0.0095,-0.0372787743898723,-0.0201758532865581));
#45830=CARTESIAN_POINT('Origin',(-0.00649999999999,-0.0372787743898623,
-0.0201758532865681));
#45831=CARTESIAN_POINT('',(-0.00949999999999,-0.0326537743470214,-0.0201758532865681));
#45832=CARTESIAN_POINT('',(-0.015,-0.0355287743470215,-0.0201758532865681));
#45833=CARTESIAN_POINT('',(0.0075,-0.035138261906077,-0.0201758532865581));
#45834=CARTESIAN_POINT('',(0.00750000000001,-0.0353335181051238,-0.0201758532865681));
#45835=CARTESIAN_POINT('Origin',(0.00600000000001,-0.0355287743898623,-0.0201758532865681));
#45836=CARTESIAN_POINT('Origin',(-0.0095,-0.0297787743898723,-0.0029758532865581));
#45837=CARTESIAN_POINT('',(-0.00949999999999,-0.0372787743898623,-0.0029758532865481));
#45838=CARTESIAN_POINT('Origin',(-0.0065,-0.0372787743898723,-0.00297585328655811));
#45839=CARTESIAN_POINT('Origin',(0.0045,-0.0297787743898723,-0.0029758532865581));
#45840=CARTESIAN_POINT('',(0.00450000000001,-0.035138261906067,-0.0029758532865481));
#45841=CARTESIAN_POINT('Origin',(0.0075,-0.035138261906077,-0.00297585328655811));
#45842=CARTESIAN_POINT('',(0.00750000000001,-0.035138261906067,-0.0029758532865481));
#45843=CARTESIAN_POINT('Origin',(0.006,-0.0355287743898723,-0.00297585328655811));
#45844=CARTESIAN_POINT('Origin',(-0.015,-0.0355287743898723,-0.0121758532865581));
#45845=CARTESIAN_POINT('',(-0.015,-0.0412787743898723,-0.00417585328655811));
#45846=CARTESIAN_POINT('Origin',(0.006,-0.0355287743898723,-0.0041758532865581));
#45847=CARTESIAN_POINT('',(0.0075,-0.035138261906077,-0.0041758532865581));
#45848=CARTESIAN_POINT('Origin',(0.00600000000001,-0.0355287743898623,-0.0041758532865581));
#45849=CARTESIAN_POINT('',(0.0075,-0.035138261906077,-0.00297585328655811));
#45850=CARTESIAN_POINT('Origin',(0.00600000000001,-0.0355287743898623,-0.0029758532865481));
#45851=CARTESIAN_POINT('',(0.00750000000001,-0.035138261906067,-0.0041758532865581));
#45852=CARTESIAN_POINT('Origin',(0.0075,-0.0297787743898723,-0.0041758532865581));
#45853=CARTESIAN_POINT('',(0.00750000000001,-0.0355287743898623,-0.0041758532865581));
#45854=CARTESIAN_POINT('',(0.00750000000001,-0.0355287743898623,-0.0029758532865481));
#45855=CARTESIAN_POINT('Origin',(-0.0095,-0.0372787743898723,-0.0041758532865581));
#45856=CARTESIAN_POINT('',(-0.0095,-0.0372787743898723,-0.0041758532865581));
#45857=CARTESIAN_POINT('',(-0.00949999999999,-0.0372787743898623,-0.0041758532865581));
#45858=CARTESIAN_POINT('',(-0.0095,-0.0372787743898723,-0.00297585328655811));
#45859=CARTESIAN_POINT('',(-0.00949999999999,-0.0372787743898623,-0.0029758532865481));
#45860=CARTESIAN_POINT('',(-0.00949999999999,-0.0372787743898623,-0.0041758532865581));
#45861=CARTESIAN_POINT('Origin',(-0.0065,-0.0372787743898723,-0.0041758532865581));
#45862=CARTESIAN_POINT('',(-0.0035,-0.0372787743898723,-0.0041758532865581));
#45863=CARTESIAN_POINT('Origin',(-0.00649999999999,-0.0372787743898623,
-0.0041758532865581));
#45864=CARTESIAN_POINT('',(-0.0035,-0.0372787743898723,-0.00297585328655811));
#45865=CARTESIAN_POINT('Origin',(-0.00649999999999,-0.0372787743898623,
-0.0029758532865481));
#45866=CARTESIAN_POINT('',(-0.00349999999999,-0.0372787743898623,-0.0041758532865581));
#45867=CARTESIAN_POINT('Origin',(-0.0035,-0.0297787743898723,-0.0041758532865581));
#45868=CARTESIAN_POINT('',(-0.00349999999999,-0.0372787743898623,-0.0041758532865581));
#45869=CARTESIAN_POINT('',(-0.00349999999999,-0.0297787743898623,-0.0029758532865481));
#45870=CARTESIAN_POINT('Origin',(-0.0035,-0.0355287743041906,-0.00297585328655811));
#45871=CARTESIAN_POINT('Origin',(-0.0035,-0.0355287743041906,-0.0041758532865581));
#50053=UNCERTAINTY_MEASURE_WITH_UNIT(LENGTH_MEASURE(1.E-5),#50082,
'DISTANCE_ACCURACY_VALUE',
'Maximum model space distance between geometric entities at asserted c
onnectivities');
#50059=UNCERTAINTY_MEASURE_WITH_UNIT(LENGTH_MEASURE(1.E-5),#50082,
'DISTANCE_ACCURACY_VALUE',
'Maximum model space distance between geometric entities at asserted c
onnectivities');
#50075=(
GEOMETRIC_REPRESENTATION_CONTEXT(3)
GLOBAL_UNCERTAINTY_ASSIGNED_CONTEXT((#50053))
GLOBAL_UNIT_ASSIGNED_CONTEXT((#50082,#50083,#50084))
REPRESENTATION_CONTEXT('','3D')
);
#50081=(
GEOMETRIC_REPRESENTATION_CONTEXT(3)
GLOBAL_UNCERTAINTY_ASSIGNED_CONTEXT((#50059))
GLOBAL_UNIT_ASSIGNED_CONTEXT((#50082,#50083,#50084))
REPRESENTATION_CONTEXT('','3D')
);
#50082=(
LENGTH_UNIT()
NAMED_UNIT(*)
SI_UNIT($,.METRE.)
);
#50083=(
NAMED_UNIT(*)
PLANE_ANGLE_UNIT()
SI_UNIT($,.RADIAN.)
);
#50084=(
NAMED_UNIT(*)
SI_UNIT($,.STERADIAN.)
SOLID_ANGLE_UNIT()
);
#50100=SHAPE_DEFINITION_REPRESENTATION(#50121,#50162);
#50121=PRODUCT_DEFINITION_SHAPE('',$,#50184);
#50162=SHAPE_REPRESENTATION('',(#10748),#50075);
#50168=PRODUCT_DEFINITION_CONTEXT('part definition',#50233,'design');
#50184=PRODUCT_DEFINITION('Silicone Heat Block Thermal Insulator',
'Silicone Heat Block Thermal Insulator',#50205,#50168);
#50205=PRODUCT_DEFINITION_FORMATION('',$,#50250);
#50233=APPLICATION_CONTEXT('Managed model based 3d engineering');
#50234=PRODUCT_CONTEXT('part definition',#50233,'mechanical');
#50250=PRODUCT('Silicone Heat Block Thermal Insulator',
'Silicone Heat Block Thermal Insulator',
'LEGAL AND USAGE DISCLAIMER: this Data/Model is provided \X2\201C\X0\A
S IS\X2\201D\X0\ for informational and representational only. It is a 
geometric approximation and is NOT engineered, certified, or guarantee
d for dimensional accuracy, exact tolerances, or production-level prec
ision. Vendor disclaims all implied warranties including fitness for a
 particular purpose. DO NOT USE FOR DIRECT PHYSICAL MANUFACTURING, AUT
OMATED PRODUCTION, OR SAFETY-CRITICAL SYSTEMS without independent engi
neering verification and resolution of any design discrepancies.',(#50234));
#50257=PRESENTATION_STYLE_ASSIGNMENT((#50264));
#50264=SURFACE_STYLE_USAGE(.BOTH.,#50271);
#50271=SURFACE_SIDE_STYLE('',(#50278));
#50278=SURFACE_STYLE_FILL_AREA(#50285);
#50285=FILL_AREA_STYLE('Opaque(137,137,137)',(#50292));
#50292=FILL_AREA_STYLE_COLOUR('Opaque(137,137,137)',#50299);
#50299=COLOUR_RGB('Opaque(137,137,137)',0.537254901960784,0.537254901960784,
0.537254901960784);
ENDSEC;
END-ISO-10303-21;
